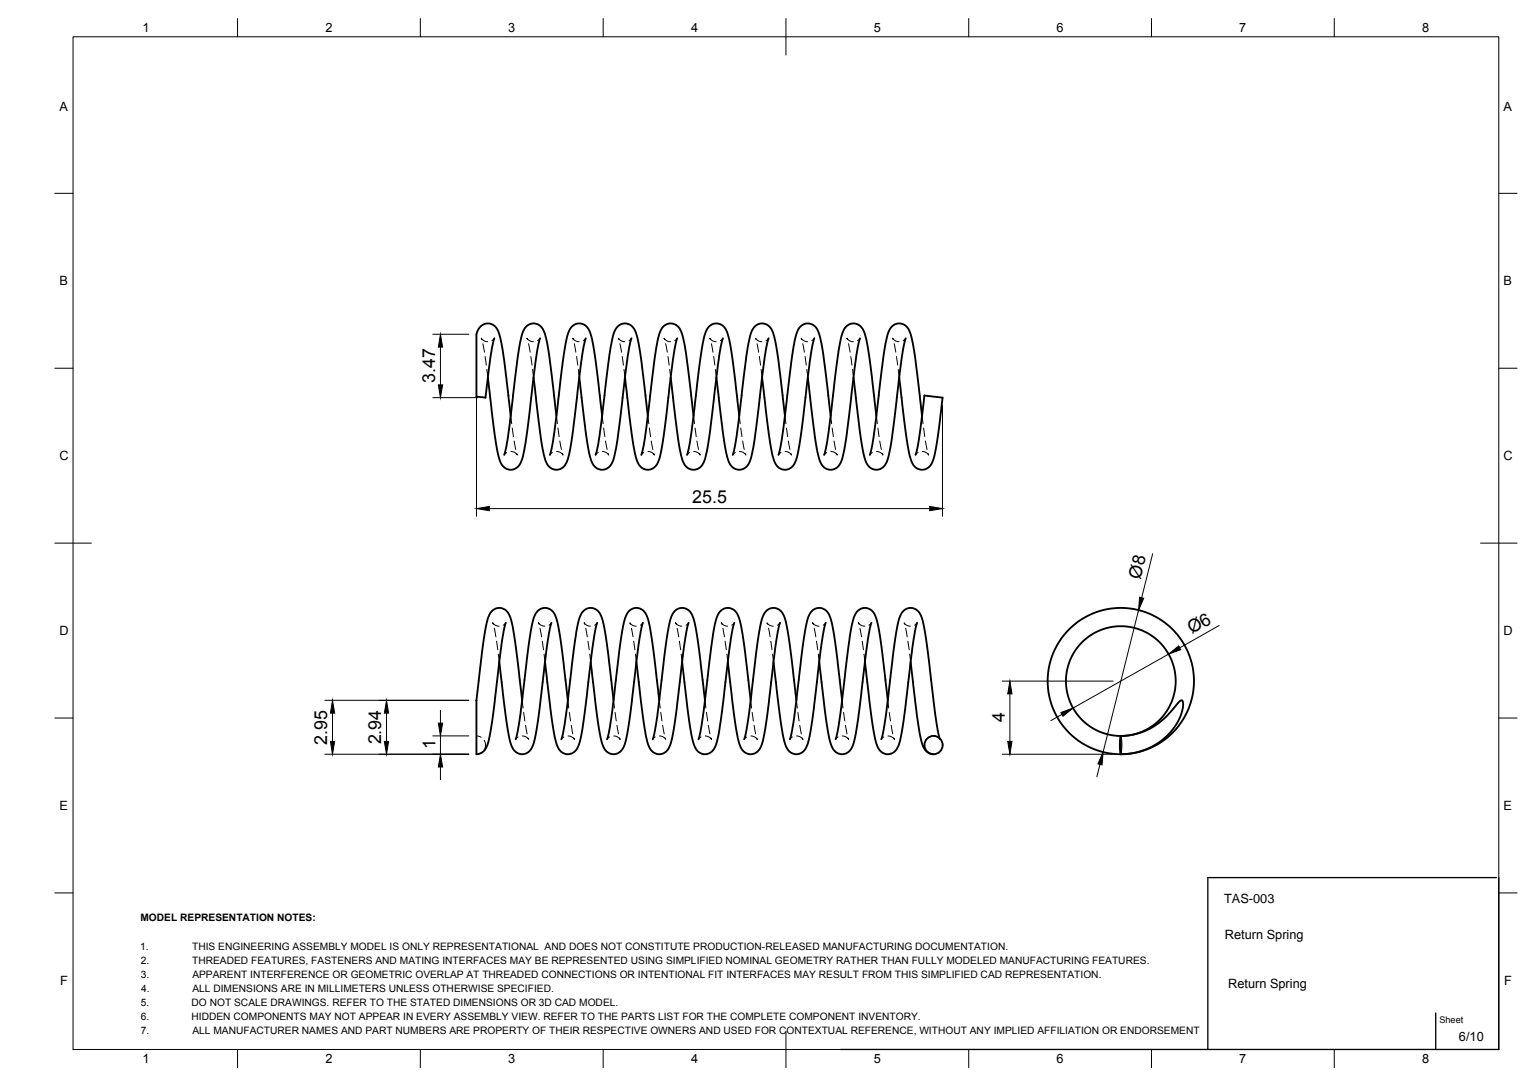
ISO-10303-21;
HEADER;
/* Generated by software containing ST-Developer
 * from STEP Tools, Inc. (www.steptools.com) 
 */

FILE_DESCRIPTION(
/* description */ ('STEP AP214'),
/* implementation_level */ '2;1');

FILE_NAME(
/* name */ 'Return Spring.step',
/* time_stamp */ '2026-11-04T19:43:37-08:00',
/* author */ (''),
/* organization */ (''),
/* preprocessor_version */ 'ST-DEVELOPER v20.2',
/* originating_system */ 'Autodesk Translation Framework v15.17.0.0',
/* authorisation */ '');

FILE_SCHEMA (('AUTOMOTIVE_DESIGN { 1 0 10303 214 3 1 1 }'));
ENDSEC;

DATA;
#10=MECHANICAL_DESIGN_GEOMETRIC_PRESENTATION_REPRESENTATION('',(#118),#7627);
#91=(
BOUNDED_CURVE()
B_SPLINE_CURVE(2,(#5252,#5253,#5254,#5255,#5256,#5257,#5258,#5259,#5260,
#5261,#5262,#5263,#5264,#5265,#5266,#5267,#5268,#5269,#5270,#5271,#5272,
#5273,#5274,#5275,#5276,#5277,#5278,#5279,#5280,#5281,#5282,#5283,#5284,
#5285,#5286,#5287,#5288,#5289,#5290,#5291,#5292,#5293,#5294,#5295,#5296,
#5297,#5298,#5299,#5300,#5301,#5302,#5303,#5304,#5305,#5306,#5307,#5308,
#5309,#5310,#5311,#5312,#5313,#5314,#5315,#5316,#5317,#5318,#5319,#5320,
#5321,#5322,#5323,#5324,#5325,#5326,#5327,#5328,#5329,#5330,#5331,#5332,
#5333,#5334,#5335,#5336,#5337,#5338,#5339,#5340,#5341,#5342,#5343,#5344,
#5345,#5346,#5347,#5348,#5349,#5350,#5351,#5352,#5353,#5354,#5355,#5356,
#5357,#5358,#5359,#5360,#5361,#5362,#5363,#5364,#5365,#5366,#5367,#5368,
#5369,#5370,#5371,#5372,#5373,#5374,#5375,#5376,#5377,#5378,#5379,#5380,
#5381,#5382,#5383,#5384,#5385,#5386,#5387,#5388,#5389,#5390,#5391,#5392,
#5393,#5394,#5395,#5396,#5397,#5398,#5399,#5400,#5401,#5402,#5403,#5404,
#5405,#5406,#5407,#5408,#5409,#5410,#5411,#5412,#5413,#5414,#5415,#5416,
#5417,#5418,#5419,#5420,#5421,#5422,#5423,#5424,#5425,#5426,#5427,#5428,
#5429,#5430,#5431,#5432,#5433,#5434,#5435,#5436,#5437,#5438,#5439,#5440,
#5441,#5442,#5443,#5444,#5445,#5446,#5447,#5448,#5449,#5450),
 .UNSPECIFIED.,.F.,.F.)
B_SPLINE_CURVE_WITH_KNOTS((3,2,2,2,2,2,2,2,2,2,2,2,2,2,2,2,2,2,2,2,2,2,
2,2,2,2,2,2,2,2,2,2,2,2,2,2,2,2,2,2,2,2,2,2,2,2,2,2,2,2,2,2,2,2,2,2,2,2,
2,2,2,2,2,2,2,2,2,2,2,2,2,2,2,2,2,2,2,2,2,2,2,2,2,2,2,2,2,2,2,2,2,2,2,2,
2,2,2,2,2,3),(0.0198656835159411,0.02,0.03,0.04,0.05,0.06,0.07,0.08,0.09,
0.1,0.11,0.12,0.13,0.14,0.15,0.16,0.17,0.18,0.19,0.2,0.21,0.22,0.23,0.24,
0.25,0.26,0.27,0.28,0.29,0.3,0.31,0.32,0.33,0.34,0.35,0.36,0.37,0.38,0.39,
0.4,0.41,0.42,0.43,0.44,0.45,0.46,0.47,0.48,0.49,0.5,0.51,0.52,0.53,0.54,
0.55,0.56,0.57,0.58,0.59,0.6,0.61,0.62,0.63,0.64,0.65,0.66,0.67,0.68,0.69,
0.7,0.71,0.72,0.73,0.74,0.75,0.76,0.77,0.78,0.79,0.8,0.81,0.82,0.83,0.84,
0.85,0.86,0.87,0.88,0.89,0.9,0.91,0.92,0.93,0.94,0.95,0.96,0.97,0.98,0.99,
1.),.UNSPECIFIED.)
CURVE()
GEOMETRIC_REPRESENTATION_ITEM()
RATIONAL_B_SPLINE_CURVE((0.998702876377649,0.999342608335117,1.,0.951056516295154,
1.,0.951056516295154,1.,0.951056516295154,1.,0.951056516295154,1.,0.951056516295154,
1.,0.951056516295154,1.,0.951056516295154,1.,0.951056516295154,1.,0.951056516295154,
1.,0.951056516295154,1.,0.951056516295154,1.,0.951056516295154,1.,0.951056516295154,
1.,0.951056516295154,1.,0.951056516295154,1.,0.951056516295154,1.,0.951056516295154,
1.,0.951056516295154,1.,0.951056516295154,1.,0.951056516295154,1.,0.951056516295154,
1.,0.951056516295154,1.,0.951056516295154,1.,0.951056516295154,1.,0.951056516295154,
1.,0.951056516295154,1.,0.951056516295154,1.,0.951056516295154,1.,0.951056516295154,
1.,0.951056516295154,1.,0.951056516295154,1.,0.951056516295154,1.,0.951056516295154,
1.,0.951056516295154,1.,0.951056516295154,1.,0.951056516295154,1.,0.951056516295154,
1.,0.951056516295154,1.,0.951056516295154,1.,0.951056516295154,1.,0.951056516295154,
1.,0.951056516295154,1.,0.951056516295154,1.,0.951056516295154,1.,0.951056516295154,
1.,0.951056516295154,1.,0.951056516295154,1.,0.951056516295154,1.,0.951056516295154,
1.,0.951056516295154,1.,0.951056516295154,1.,0.951056516295154,1.,0.951056516295154,
1.,0.951056516295154,1.,0.951056516295154,1.,0.951056516295154,1.,0.951056516295154,
1.,0.951056516295154,1.,0.951056516295154,1.,0.951056516295154,1.,0.951056516295154,
1.,0.951056516295154,1.,0.951056516295154,1.,0.951056516295154,1.,0.951056516295154,
1.,0.951056516295154,1.,0.951056516295154,1.,0.951056516295154,1.,0.951056516295154,
1.,0.951056516295154,1.,0.951056516295154,1.,0.951056516295154,1.,0.951056516295154,
1.,0.951056516295154,1.,0.951056516295154,1.,0.951056516295154,1.,0.951056516295154,
1.,0.951056516295154,1.,0.951056516295154,1.,0.951056516295154,1.,0.951056516295154,
1.,0.951056516295154,1.,0.951056516295154,1.,0.951056516295154,1.,0.951056516295154,
1.,0.951056516295154,1.,0.951056516295154,1.,0.951056516295154,1.,0.951056516295154,
1.,0.951056516295154,1.,0.951056516295154,1.,0.951056516295154,1.,0.951056516295154,
1.,0.951056516295154,1.,0.951056516295154,1.,0.951056516295154,1.,0.951056516295154,
1.,0.951056516295154,1.))
REPRESENTATION_ITEM('')
);
#92=(
BOUNDED_CURVE()
B_SPLINE_CURVE(2,(#5454,#5455,#5456,#5457,#5458,#5459,#5460,#5461,#5462,
#5463,#5464,#5465,#5466,#5467,#5468,#5469,#5470,#5471,#5472,#5473,#5474,
#5475,#5476,#5477,#5478,#5479,#5480,#5481,#5482,#5483,#5484,#5485,#5486,
#5487,#5488,#5489,#5490,#5491,#5492,#5493,#5494,#5495,#5496,#5497,#5498,
#5499,#5500,#5501,#5502,#5503,#5504,#5505,#5506,#5507,#5508,#5509,#5510,
#5511,#5512,#5513,#5514,#5515,#5516,#5517,#5518,#5519,#5520,#5521,#5522,
#5523,#5524,#5525,#5526,#5527,#5528,#5529,#5530,#5531,#5532,#5533,#5534,
#5535,#5536,#5537,#5538,#5539,#5540,#5541,#5542,#5543,#5544,#5545,#5546,
#5547,#5548,#5549,#5550,#5551,#5552,#5553,#5554,#5555,#5556,#5557,#5558,
#5559,#5560,#5561,#5562,#5563,#5564,#5565,#5566,#5567,#5568,#5569,#5570,
#5571,#5572,#5573,#5574,#5575,#5576,#5577,#5578,#5579,#5580,#5581,#5582,
#5583,#5584,#5585,#5586,#5587,#5588,#5589,#5590,#5591,#5592,#5593,#5594,
#5595,#5596,#5597,#5598,#5599,#5600,#5601,#5602,#5603,#5604,#5605,#5606,
#5607,#5608,#5609,#5610,#5611,#5612,#5613,#5614,#5615,#5616,#5617,#5618,
#5619,#5620,#5621,#5622,#5623,#5624,#5625,#5626,#5627,#5628,#5629,#5630,
#5631,#5632,#5633,#5634,#5635,#5636,#5637,#5638,#5639,#5640,#5641,#5642,
#5643,#5644,#5645,#5646,#5647,#5648,#5649,#5650,#5651,#5652,#5653,#5654),
 .UNSPECIFIED.,.F.,.F.)
B_SPLINE_CURVE_WITH_KNOTS((3,2,2,2,2,2,2,2,2,2,2,2,2,2,2,2,2,2,2,2,2,2,
2,2,2,2,2,2,2,2,2,2,2,2,2,2,2,2,2,2,2,2,2,2,2,2,2,2,2,2,2,2,2,2,2,2,2,2,
2,2,2,2,2,2,2,2,2,2,2,2,2,2,2,2,2,2,2,2,2,2,2,2,2,2,2,2,2,2,2,2,2,2,2,2,
2,2,2,2,2,2,3),(0.,0.01,0.02,0.03,0.04,0.05,0.06,0.07,0.08,0.09,0.1,0.11,
0.12,0.13,0.14,0.15,0.16,0.17,0.18,0.19,0.2,0.21,0.22,0.23,0.24,0.25,0.26,
0.27,0.28,0.29,0.3,0.31,0.32,0.33,0.34,0.35,0.36,0.37,0.38,0.39,0.4,0.41,
0.42,0.43,0.44,0.45,0.46,0.47,0.48,0.49,0.5,0.51,0.52,0.53,0.54,0.55,0.56,
0.57,0.58,0.59,0.6,0.61,0.62,0.63,0.64,0.65,0.66,0.67,0.68,0.69,0.7,0.71,
0.72,0.73,0.74,0.75,0.76,0.77,0.78,0.79,0.8,0.81,0.82,0.83,0.84,0.85,0.86,
0.87,0.88,0.89,0.9,0.91,0.92,0.93,0.94,0.95,0.96,0.97,0.98,0.99,1.),
 .UNSPECIFIED.)
CURVE()
GEOMETRIC_REPRESENTATION_ITEM()
RATIONAL_B_SPLINE_CURVE((1.,0.951056516295154,1.,0.951056516295154,1.,0.951056516295154,
1.,0.951056516295154,1.,0.951056516295154,1.,0.951056516295154,1.,0.951056516295154,
1.,0.951056516295154,1.,0.951056516295154,1.,0.951056516295154,1.,0.951056516295154,
1.,0.951056516295154,1.,0.951056516295154,1.,0.951056516295154,1.,0.951056516295154,
1.,0.951056516295154,1.,0.951056516295154,1.,0.951056516295154,1.,0.951056516295154,
1.,0.951056516295154,1.,0.951056516295154,1.,0.951056516295154,1.,0.951056516295154,
1.,0.951056516295154,1.,0.951056516295154,1.,0.951056516295154,1.,0.951056516295154,
1.,0.951056516295154,1.,0.951056516295154,1.,0.951056516295154,1.,0.951056516295154,
1.,0.951056516295154,1.,0.951056516295154,1.,0.951056516295154,1.,0.951056516295154,
1.,0.951056516295154,1.,0.951056516295154,1.,0.951056516295154,1.,0.951056516295154,
1.,0.951056516295154,1.,0.951056516295154,1.,0.951056516295154,1.,0.951056516295154,
1.,0.951056516295154,1.,0.951056516295154,1.,0.951056516295154,1.,0.951056516295154,
1.,0.951056516295154,1.,0.951056516295154,1.,0.951056516295154,1.,0.951056516295154,
1.,0.951056516295154,1.,0.951056516295154,1.,0.951056516295154,1.,0.951056516295154,
1.,0.951056516295154,1.,0.951056516295154,1.,0.951056516295154,1.,0.951056516295154,
1.,0.951056516295154,1.,0.951056516295154,1.,0.951056516295154,1.,0.951056516295154,
1.,0.951056516295154,1.,0.951056516295154,1.,0.951056516295154,1.,0.951056516295154,
1.,0.951056516295154,1.,0.951056516295154,1.,0.951056516295154,1.,0.951056516295154,
1.,0.951056516295154,1.,0.951056516295154,1.,0.951056516295154,1.,0.951056516295154,
1.,0.951056516295154,1.,0.951056516295154,1.,0.951056516295154,1.,0.951056516295154,
1.,0.951056516295154,1.,0.951056516295154,1.,0.951056516295154,1.,0.951056516295154,
1.,0.951056516295154,1.,0.951056516295154,1.,0.951056516295154,1.,0.951056516295154,
1.,0.951056516295154,1.,0.951056516295154,1.,0.951056516295154,1.,0.951056516295154,
1.,0.951056516295154,1.,0.951056516295154,1.,0.951056516295154,1.,0.951056516295154,
1.,0.951056516295154,1.,0.951056516295154,1.,0.951056516295154,1.,0.951056516295154,
1.,0.951056516295154,1.))
REPRESENTATION_ITEM('')
);
#93=B_SPLINE_CURVE_WITH_KNOTS('',3,(#5233,#5234,#5235,#5236,#5237,#5238,
#5239,#5240,#5241,#5242,#5243,#5244,#5245,#5246,#5247,#5248,#5249,#5250),
 .UNSPECIFIED.,.F.,.F.,(4,2,2,2,2,2,2,2,4),(1.00001181076875E-6,0.00157652680691075,
0.00330831465659758,0.00743558655671621,0.0176553842502255,0.0434588790338826,
0.0717527150596022,0.0885002828939342,0.104340792550165),.UNSPECIFIED.);
#94=B_SPLINE_CURVE_WITH_KNOTS('',3,(#7069,#7070,#7071,#7072,#7073,#7074,
#7075,#7076,#7077,#7078,#7079,#7080,#7081,#7082,#7083,#7084,#7085,#7086),
 .UNSPECIFIED.,.F.,.F.,(4,2,2,2,2,2,2,2,4),(0.,0.132188814767311,0.250674887289718,
0.391272166110131,0.552836235371939,0.655950520994649,0.689957274574409,
0.701859173270786,0.711834218003037),.UNSPECIFIED.);
#95=(
BOUNDED_SURFACE()
B_SPLINE_SURFACE(3,2,((#3824,#3825,#3826,#3827,#3828,#3829,#3830,#3831,
#3832,#3833,#3834,#3835,#3836,#3837,#3838,#3839,#3840,#3841,#3842,#3843,
#3844,#3845,#3846,#3847,#3848,#3849,#3850,#3851,#3852,#3853,#3854,#3855,
#3856,#3857,#3858,#3859,#3860,#3861,#3862,#3863,#3864,#3865,#3866,#3867,
#3868,#3869,#3870,#3871,#3872,#3873,#3874,#3875,#3876,#3877,#3878,#3879,
#3880,#3881,#3882,#3883,#3884,#3885,#3886,#3887,#3888,#3889,#3890,#3891,
#3892,#3893,#3894,#3895,#3896,#3897,#3898,#3899,#3900,#3901,#3902,#3903,
#3904,#3905,#3906,#3907,#3908,#3909,#3910,#3911,#3912,#3913,#3914,#3915,
#3916,#3917,#3918,#3919,#3920,#3921,#3922,#3923,#3924,#3925,#3926,#3927,
#3928,#3929,#3930,#3931,#3932,#3933,#3934,#3935,#3936,#3937,#3938,#3939,
#3940,#3941,#3942,#3943,#3944,#3945,#3946,#3947,#3948,#3949,#3950,#3951,
#3952,#3953,#3954,#3955,#3956,#3957,#3958,#3959,#3960,#3961,#3962,#3963,
#3964,#3965,#3966,#3967,#3968,#3969,#3970,#3971,#3972,#3973,#3974,#3975,
#3976,#3977,#3978,#3979,#3980,#3981,#3982,#3983,#3984,#3985,#3986,#3987,
#3988,#3989,#3990,#3991,#3992,#3993,#3994,#3995,#3996,#3997,#3998,#3999,
#4000,#4001,#4002,#4003,#4004,#4005,#4006,#4007,#4008,#4009,#4010,#4011,
#4012,#4013,#4014,#4015,#4016,#4017,#4018,#4019,#4020,#4021,#4022,#4023,
#4024),(#4025,#4026,#4027,#4028,#4029,#4030,#4031,#4032,#4033,#4034,#4035,
#4036,#4037,#4038,#4039,#4040,#4041,#4042,#4043,#4044,#4045,#4046,#4047,
#4048,#4049,#4050,#4051,#4052,#4053,#4054,#4055,#4056,#4057,#4058,#4059,
#4060,#4061,#4062,#4063,#4064,#4065,#4066,#4067,#4068,#4069,#4070,#4071,
#4072,#4073,#4074,#4075,#4076,#4077,#4078,#4079,#4080,#4081,#4082,#4083,
#4084,#4085,#4086,#4087,#4088,#4089,#4090,#4091,#4092,#4093,#4094,#4095,
#4096,#4097,#4098,#4099,#4100,#4101,#4102,#4103,#4104,#4105,#4106,#4107,
#4108,#4109,#4110,#4111,#4112,#4113,#4114,#4115,#4116,#4117,#4118,#4119,
#4120,#4121,#4122,#4123,#4124,#4125,#4126,#4127,#4128,#4129,#4130,#4131,
#4132,#4133,#4134,#4135,#4136,#4137,#4138,#4139,#4140,#4141,#4142,#4143,
#4144,#4145,#4146,#4147,#4148,#4149,#4150,#4151,#4152,#4153,#4154,#4155,
#4156,#4157,#4158,#4159,#4160,#4161,#4162,#4163,#4164,#4165,#4166,#4167,
#4168,#4169,#4170,#4171,#4172,#4173,#4174,#4175,#4176,#4177,#4178,#4179,
#4180,#4181,#4182,#4183,#4184,#4185,#4186,#4187,#4188,#4189,#4190,#4191,
#4192,#4193,#4194,#4195,#4196,#4197,#4198,#4199,#4200,#4201,#4202,#4203,
#4204,#4205,#4206,#4207,#4208,#4209,#4210,#4211,#4212,#4213,#4214,#4215,
#4216,#4217,#4218,#4219,#4220,#4221,#4222,#4223,#4224,#4225),(#4226,#4227,
#4228,#4229,#4230,#4231,#4232,#4233,#4234,#4235,#4236,#4237,#4238,#4239,
#4240,#4241,#4242,#4243,#4244,#4245,#4246,#4247,#4248,#4249,#4250,#4251,
#4252,#4253,#4254,#4255,#4256,#4257,#4258,#4259,#4260,#4261,#4262,#4263,
#4264,#4265,#4266,#4267,#4268,#4269,#4270,#4271,#4272,#4273,#4274,#4275,
#4276,#4277,#4278,#4279,#4280,#4281,#4282,#4283,#4284,#4285,#4286,#4287,
#4288,#4289,#4290,#4291,#4292,#4293,#4294,#4295,#4296,#4297,#4298,#4299,
#4300,#4301,#4302,#4303,#4304,#4305,#4306,#4307,#4308,#4309,#4310,#4311,
#4312,#4313,#4314,#4315,#4316,#4317,#4318,#4319,#4320,#4321,#4322,#4323,
#4324,#4325,#4326,#4327,#4328,#4329,#4330,#4331,#4332,#4333,#4334,#4335,
#4336,#4337,#4338,#4339,#4340,#4341,#4342,#4343,#4344,#4345,#4346,#4347,
#4348,#4349,#4350,#4351,#4352,#4353,#4354,#4355,#4356,#4357,#4358,#4359,
#4360,#4361,#4362,#4363,#4364,#4365,#4366,#4367,#4368,#4369,#4370,#4371,
#4372,#4373,#4374,#4375,#4376,#4377,#4378,#4379,#4380,#4381,#4382,#4383,
#4384,#4385,#4386,#4387,#4388,#4389,#4390,#4391,#4392,#4393,#4394,#4395,
#4396,#4397,#4398,#4399,#4400,#4401,#4402,#4403,#4404,#4405,#4406,#4407,
#4408,#4409,#4410,#4411,#4412,#4413,#4414,#4415,#4416,#4417,#4418,#4419,
#4420,#4421,#4422,#4423,#4424,#4425,#4426),(#4427,#4428,#4429,#4430,#4431,
#4432,#4433,#4434,#4435,#4436,#4437,#4438,#4439,#4440,#4441,#4442,#4443,
#4444,#4445,#4446,#4447,#4448,#4449,#4450,#4451,#4452,#4453,#4454,#4455,
#4456,#4457,#4458,#4459,#4460,#4461,#4462,#4463,#4464,#4465,#4466,#4467,
#4468,#4469,#4470,#4471,#4472,#4473,#4474,#4475,#4476,#4477,#4478,#4479,
#4480,#4481,#4482,#4483,#4484,#4485,#4486,#4487,#4488,#4489,#4490,#4491,
#4492,#4493,#4494,#4495,#4496,#4497,#4498,#4499,#4500,#4501,#4502,#4503,
#4504,#4505,#4506,#4507,#4508,#4509,#4510,#4511,#4512,#4513,#4514,#4515,
#4516,#4517,#4518,#4519,#4520,#4521,#4522,#4523,#4524,#4525,#4526,#4527,
#4528,#4529,#4530,#4531,#4532,#4533,#4534,#4535,#4536,#4537,#4538,#4539,
#4540,#4541,#4542,#4543,#4544,#4545,#4546,#4547,#4548,#4549,#4550,#4551,
#4552,#4553,#4554,#4555,#4556,#4557,#4558,#4559,#4560,#4561,#4562,#4563,
#4564,#4565,#4566,#4567,#4568,#4569,#4570,#4571,#4572,#4573,#4574,#4575,
#4576,#4577,#4578,#4579,#4580,#4581,#4582,#4583,#4584,#4585,#4586,#4587,
#4588,#4589,#4590,#4591,#4592,#4593,#4594,#4595,#4596,#4597,#4598,#4599,
#4600,#4601,#4602,#4603,#4604,#4605,#4606,#4607,#4608,#4609,#4610,#4611,
#4612,#4613,#4614,#4615,#4616,#4617,#4618,#4619,#4620,#4621,#4622,#4623,
#4624,#4625,#4626,#4627),(#4628,#4629,#4630,#4631,#4632,#4633,#4634,#4635,
#4636,#4637,#4638,#4639,#4640,#4641,#4642,#4643,#4644,#4645,#4646,#4647,
#4648,#4649,#4650,#4651,#4652,#4653,#4654,#4655,#4656,#4657,#4658,#4659,
#4660,#4661,#4662,#4663,#4664,#4665,#4666,#4667,#4668,#4669,#4670,#4671,
#4672,#4673,#4674,#4675,#4676,#4677,#4678,#4679,#4680,#4681,#4682,#4683,
#4684,#4685,#4686,#4687,#4688,#4689,#4690,#4691,#4692,#4693,#4694,#4695,
#4696,#4697,#4698,#4699,#4700,#4701,#4702,#4703,#4704,#4705,#4706,#4707,
#4708,#4709,#4710,#4711,#4712,#4713,#4714,#4715,#4716,#4717,#4718,#4719,
#4720,#4721,#4722,#4723,#4724,#4725,#4726,#4727,#4728,#4729,#4730,#4731,
#4732,#4733,#4734,#4735,#4736,#4737,#4738,#4739,#4740,#4741,#4742,#4743,
#4744,#4745,#4746,#4747,#4748,#4749,#4750,#4751,#4752,#4753,#4754,#4755,
#4756,#4757,#4758,#4759,#4760,#4761,#4762,#4763,#4764,#4765,#4766,#4767,
#4768,#4769,#4770,#4771,#4772,#4773,#4774,#4775,#4776,#4777,#4778,#4779,
#4780,#4781,#4782,#4783,#4784,#4785,#4786,#4787,#4788,#4789,#4790,#4791,
#4792,#4793,#4794,#4795,#4796,#4797,#4798,#4799,#4800,#4801,#4802,#4803,
#4804,#4805,#4806,#4807,#4808,#4809,#4810,#4811,#4812,#4813,#4814,#4815,
#4816,#4817,#4818,#4819,#4820,#4821,#4822,#4823,#4824,#4825,#4826,#4827,
#4828),(#4829,#4830,#4831,#4832,#4833,#4834,#4835,#4836,#4837,#4838,#4839,
#4840,#4841,#4842,#4843,#4844,#4845,#4846,#4847,#4848,#4849,#4850,#4851,
#4852,#4853,#4854,#4855,#4856,#4857,#4858,#4859,#4860,#4861,#4862,#4863,
#4864,#4865,#4866,#4867,#4868,#4869,#4870,#4871,#4872,#4873,#4874,#4875,
#4876,#4877,#4878,#4879,#4880,#4881,#4882,#4883,#4884,#4885,#4886,#4887,
#4888,#4889,#4890,#4891,#4892,#4893,#4894,#4895,#4896,#4897,#4898,#4899,
#4900,#4901,#4902,#4903,#4904,#4905,#4906,#4907,#4908,#4909,#4910,#4911,
#4912,#4913,#4914,#4915,#4916,#4917,#4918,#4919,#4920,#4921,#4922,#4923,
#4924,#4925,#4926,#4927,#4928,#4929,#4930,#4931,#4932,#4933,#4934,#4935,
#4936,#4937,#4938,#4939,#4940,#4941,#4942,#4943,#4944,#4945,#4946,#4947,
#4948,#4949,#4950,#4951,#4952,#4953,#4954,#4955,#4956,#4957,#4958,#4959,
#4960,#4961,#4962,#4963,#4964,#4965,#4966,#4967,#4968,#4969,#4970,#4971,
#4972,#4973,#4974,#4975,#4976,#4977,#4978,#4979,#4980,#4981,#4982,#4983,
#4984,#4985,#4986,#4987,#4988,#4989,#4990,#4991,#4992,#4993,#4994,#4995,
#4996,#4997,#4998,#4999,#5000,#5001,#5002,#5003,#5004,#5005,#5006,#5007,
#5008,#5009,#5010,#5011,#5012,#5013,#5014,#5015,#5016,#5017,#5018,#5019,
#5020,#5021,#5022,#5023,#5024,#5025,#5026,#5027,#5028,#5029),(#5030,#5031,
#5032,#5033,#5034,#5035,#5036,#5037,#5038,#5039,#5040,#5041,#5042,#5043,
#5044,#5045,#5046,#5047,#5048,#5049,#5050,#5051,#5052,#5053,#5054,#5055,
#5056,#5057,#5058,#5059,#5060,#5061,#5062,#5063,#5064,#5065,#5066,#5067,
#5068,#5069,#5070,#5071,#5072,#5073,#5074,#5075,#5076,#5077,#5078,#5079,
#5080,#5081,#5082,#5083,#5084,#5085,#5086,#5087,#5088,#5089,#5090,#5091,
#5092,#5093,#5094,#5095,#5096,#5097,#5098,#5099,#5100,#5101,#5102,#5103,
#5104,#5105,#5106,#5107,#5108,#5109,#5110,#5111,#5112,#5113,#5114,#5115,
#5116,#5117,#5118,#5119,#5120,#5121,#5122,#5123,#5124,#5125,#5126,#5127,
#5128,#5129,#5130,#5131,#5132,#5133,#5134,#5135,#5136,#5137,#5138,#5139,
#5140,#5141,#5142,#5143,#5144,#5145,#5146,#5147,#5148,#5149,#5150,#5151,
#5152,#5153,#5154,#5155,#5156,#5157,#5158,#5159,#5160,#5161,#5162,#5163,
#5164,#5165,#5166,#5167,#5168,#5169,#5170,#5171,#5172,#5173,#5174,#5175,
#5176,#5177,#5178,#5179,#5180,#5181,#5182,#5183,#5184,#5185,#5186,#5187,
#5188,#5189,#5190,#5191,#5192,#5193,#5194,#5195,#5196,#5197,#5198,#5199,
#5200,#5201,#5202,#5203,#5204,#5205,#5206,#5207,#5208,#5209,#5210,#5211,
#5212,#5213,#5214,#5215,#5216,#5217,#5218,#5219,#5220,#5221,#5222,#5223,
#5224,#5225,#5226,#5227,#5228,#5229,#5230)),.UNSPECIFIED.,.T.,.F.,.F.)
B_SPLINE_SURFACE_WITH_KNOTS((4,3,4),(3,2,2,2,2,2,2,2,2,2,2,2,2,2,2,2,2,
2,2,2,2,2,2,2,2,2,2,2,2,2,2,2,2,2,2,2,2,2,2,2,2,2,2,2,2,2,2,2,2,2,2,2,2,
2,2,2,2,2,2,2,2,2,2,2,2,2,2,2,2,2,2,2,2,2,2,2,2,2,2,2,2,2,2,2,2,2,2,2,2,
2,2,2,2,2,2,2,2,2,2,2,3),(0.,0.5,1.),(0.,0.01,0.02,0.03,0.04,0.05,0.06,
0.07,0.08,0.09,0.1,0.11,0.12,0.13,0.14,0.15,0.16,0.17,0.18,0.19,0.2,0.21,
0.22,0.23,0.24,0.25,0.26,0.27,0.28,0.29,0.3,0.31,0.32,0.33,0.34,0.35,0.36,
0.37,0.38,0.39,0.4,0.41,0.42,0.43,0.44,0.45,0.46,0.47,0.48,0.49,0.5,0.51,
0.52,0.53,0.54,0.55,0.56,0.57,0.58,0.59,0.6,0.61,0.62,0.63,0.64,0.65,0.66,
0.67,0.68,0.69,0.7,0.71,0.72,0.73,0.74,0.75,0.76,0.77,0.78,0.79,0.8,0.81,
0.82,0.83,0.84,0.85,0.86,0.87,0.88,0.89,0.9,0.91,0.92,0.93,0.94,0.95,0.96,
0.97,0.98,0.99,1.),.UNSPECIFIED.)
GEOMETRIC_REPRESENTATION_ITEM()
RATIONAL_B_SPLINE_SURFACE(((1.,0.951056516295154,1.,0.951056516295154,1.,
0.951056516295154,1.,0.951056516295154,1.,0.951056516295154,1.,0.951056516295154,
1.,0.951056516295154,1.,0.951056516295154,1.,0.951056516295154,1.,0.951056516295154,
1.,0.951056516295154,1.,0.951056516295154,1.,0.951056516295154,1.,0.951056516295154,
1.,0.951056516295154,1.,0.951056516295154,1.,0.951056516295154,1.,0.951056516295154,
1.,0.951056516295154,1.,0.951056516295154,1.,0.951056516295154,1.,0.951056516295154,
1.,0.951056516295154,1.,0.951056516295154,1.,0.951056516295154,1.,0.951056516295154,
1.,0.951056516295154,1.,0.951056516295154,1.,0.951056516295154,1.,0.951056516295154,
1.,0.951056516295154,1.,0.951056516295154,1.,0.951056516295154,1.,0.951056516295154,
1.,0.951056516295154,1.,0.951056516295154,1.,0.951056516295154,1.,0.951056516295154,
1.,0.951056516295154,1.,0.951056516295154,1.,0.951056516295154,1.,0.951056516295154,
1.,0.951056516295154,1.,0.951056516295154,1.,0.951056516295154,1.,0.951056516295154,
1.,0.951056516295154,1.,0.951056516295154,1.,0.951056516295154,1.,0.951056516295154,
1.,0.951056516295154,1.,0.951056516295154,1.,0.951056516295154,1.,0.951056516295154,
1.,0.951056516295154,1.,0.951056516295154,1.,0.951056516295154,1.,0.951056516295154,
1.,0.951056516295154,1.,0.951056516295154,1.,0.951056516295154,1.,0.951056516295154,
1.,0.951056516295154,1.,0.951056516295154,1.,0.951056516295154,1.,0.951056516295154,
1.,0.951056516295154,1.,0.951056516295154,1.,0.951056516295154,1.,0.951056516295154,
1.,0.951056516295154,1.,0.951056516295154,1.,0.951056516295154,1.,0.951056516295154,
1.,0.951056516295154,1.,0.951056516295154,1.,0.951056516295154,1.,0.951056516295154,
1.,0.951056516295154,1.,0.951056516295154,1.,0.951056516295154,1.,0.951056516295154,
1.,0.951056516295154,1.,0.951056516295154,1.,0.951056516295154,1.,0.951056516295154,
1.,0.951056516295154,1.,0.951056516295154,1.,0.951056516295154,1.,0.951056516295154,
1.,0.951056516295154,1.,0.951056516295154,1.,0.951056516295154,1.,0.951056516295154,
1.,0.951056516295154,1.,0.951056516295154,1.,0.951056516295154,1.,0.951056516295154,
1.,0.951056516295154,1.,0.951056516295154,1.),(0.333333333333333,0.317018838765051,
0.333333333333333,0.317018838765051,0.333333333333333,0.317018838765051,
0.333333333333333,0.317018838765051,0.333333333333333,0.317018838765051,
0.333333333333333,0.317018838765051,0.333333333333333,0.317018838765051,
0.333333333333333,0.317018838765051,0.333333333333333,0.317018838765051,
0.333333333333333,0.317018838765051,0.333333333333333,0.317018838765051,
0.333333333333333,0.317018838765051,0.333333333333333,0.317018838765051,
0.333333333333333,0.317018838765051,0.333333333333333,0.317018838765051,
0.333333333333333,0.317018838765051,0.333333333333333,0.317018838765051,
0.333333333333333,0.317018838765051,0.333333333333333,0.317018838765051,
0.333333333333333,0.317018838765051,0.333333333333333,0.317018838765051,
0.333333333333333,0.317018838765051,0.333333333333333,0.317018838765051,
0.333333333333333,0.317018838765051,0.333333333333333,0.317018838765051,
0.333333333333333,0.317018838765051,0.333333333333333,0.317018838765051,
0.333333333333333,0.317018838765051,0.333333333333333,0.317018838765051,
0.333333333333333,0.317018838765051,0.333333333333333,0.317018838765051,
0.333333333333333,0.317018838765051,0.333333333333333,0.317018838765051,
0.333333333333333,0.317018838765051,0.333333333333333,0.317018838765051,
0.333333333333333,0.317018838765051,0.333333333333333,0.317018838765051,
0.333333333333333,0.317018838765051,0.333333333333333,0.317018838765051,
0.333333333333333,0.317018838765051,0.333333333333333,0.317018838765051,
0.333333333333333,0.317018838765051,0.333333333333333,0.317018838765051,
0.333333333333333,0.317018838765051,0.333333333333333,0.317018838765051,
0.333333333333333,0.317018838765051,0.333333333333333,0.317018838765051,
0.333333333333333,0.317018838765051,0.333333333333333,0.317018838765051,
0.333333333333333,0.317018838765051,0.333333333333333,0.317018838765051,
0.333333333333333,0.317018838765051,0.333333333333333,0.317018838765051,
0.333333333333333,0.317018838765051,0.333333333333333,0.317018838765051,
0.333333333333333,0.317018838765051,0.333333333333333,0.317018838765051,
0.333333333333333,0.317018838765051,0.333333333333333,0.317018838765051,
0.333333333333333,0.317018838765051,0.333333333333333,0.317018838765051,
0.333333333333333,0.317018838765051,0.333333333333333,0.317018838765051,
0.333333333333333,0.317018838765051,0.333333333333333,0.317018838765051,
0.333333333333333,0.317018838765051,0.333333333333333,0.317018838765051,
0.333333333333333,0.317018838765051,0.333333333333333,0.317018838765051,
0.333333333333333,0.317018838765051,0.333333333333333,0.317018838765051,
0.333333333333333,0.317018838765051,0.333333333333333,0.317018838765051,
0.333333333333333,0.317018838765051,0.333333333333333,0.317018838765051,
0.333333333333333,0.317018838765051,0.333333333333333,0.317018838765051,
0.333333333333333,0.317018838765051,0.333333333333333,0.317018838765051,
0.333333333333333,0.317018838765051,0.333333333333333,0.317018838765051,
0.333333333333333,0.317018838765051,0.333333333333333,0.317018838765051,
0.333333333333333,0.317018838765051,0.333333333333333,0.317018838765051,
0.333333333333333,0.317018838765051,0.333333333333333,0.317018838765051,
0.333333333333333,0.317018838765051,0.333333333333333,0.317018838765051,
0.333333333333333,0.317018838765051,0.333333333333333,0.317018838765051,
0.333333333333333,0.317018838765051,0.333333333333333,0.317018838765051,
0.333333333333333,0.317018838765051,0.333333333333333,0.317018838765051,
0.333333333333333,0.317018838765051,0.333333333333333,0.317018838765051,
0.333333333333333,0.317018838765051,0.333333333333333,0.317018838765051,
0.333333333333333,0.317018838765051,0.333333333333333),(0.333333333333333,
0.317018838765051,0.333333333333333,0.317018838765051,0.333333333333333,
0.317018838765051,0.333333333333333,0.317018838765051,0.333333333333333,
0.317018838765051,0.333333333333333,0.317018838765051,0.333333333333333,
0.317018838765051,0.333333333333333,0.317018838765051,0.333333333333333,
0.317018838765051,0.333333333333333,0.317018838765051,0.333333333333333,
0.317018838765051,0.333333333333333,0.317018838765051,0.333333333333333,
0.317018838765051,0.333333333333333,0.317018838765051,0.333333333333333,
0.317018838765051,0.333333333333333,0.317018838765051,0.333333333333333,
0.317018838765051,0.333333333333333,0.317018838765051,0.333333333333333,
0.317018838765051,0.333333333333333,0.317018838765051,0.333333333333333,
0.317018838765051,0.333333333333333,0.317018838765051,0.333333333333333,
0.317018838765051,0.333333333333333,0.317018838765051,0.333333333333333,
0.317018838765051,0.333333333333333,0.317018838765051,0.333333333333333,
0.317018838765051,0.333333333333333,0.317018838765051,0.333333333333333,
0.317018838765051,0.333333333333333,0.317018838765051,0.333333333333333,
0.317018838765051,0.333333333333333,0.317018838765051,0.333333333333333,
0.317018838765051,0.333333333333333,0.317018838765051,0.333333333333333,
0.317018838765051,0.333333333333333,0.317018838765051,0.333333333333333,
0.317018838765051,0.333333333333333,0.317018838765051,0.333333333333333,
0.317018838765051,0.333333333333333,0.317018838765051,0.333333333333333,
0.317018838765051,0.333333333333333,0.317018838765051,0.333333333333333,
0.317018838765051,0.333333333333333,0.317018838765051,0.333333333333333,
0.317018838765051,0.333333333333333,0.317018838765051,0.333333333333333,
0.317018838765051,0.333333333333333,0.317018838765051,0.333333333333333,
0.317018838765051,0.333333333333333,0.317018838765051,0.333333333333333,
0.317018838765051,0.333333333333333,0.317018838765051,0.333333333333333,
0.317018838765051,0.333333333333333,0.317018838765051,0.333333333333333,
0.317018838765051,0.333333333333333,0.317018838765051,0.333333333333333,
0.317018838765051,0.333333333333333,0.317018838765051,0.333333333333333,
0.317018838765051,0.333333333333333,0.317018838765051,0.333333333333333,
0.317018838765051,0.333333333333333,0.317018838765051,0.333333333333333,
0.317018838765051,0.333333333333333,0.317018838765051,0.333333333333333,
0.317018838765051,0.333333333333333,0.317018838765051,0.333333333333333,
0.317018838765051,0.333333333333333,0.317018838765051,0.333333333333333,
0.317018838765051,0.333333333333333,0.317018838765051,0.333333333333333,
0.317018838765051,0.333333333333333,0.317018838765051,0.333333333333333,
0.317018838765051,0.333333333333333,0.317018838765051,0.333333333333333,
0.317018838765051,0.333333333333333,0.317018838765051,0.333333333333333,
0.317018838765051,0.333333333333333,0.317018838765051,0.333333333333333,
0.317018838765051,0.333333333333333,0.317018838765051,0.333333333333333,
0.317018838765051,0.333333333333333,0.317018838765051,0.333333333333333,
0.317018838765051,0.333333333333333,0.317018838765051,0.333333333333333,
0.317018838765051,0.333333333333333,0.317018838765051,0.333333333333333,
0.317018838765051,0.333333333333333,0.317018838765051,0.333333333333333,
0.317018838765051,0.333333333333333,0.317018838765051,0.333333333333333,
0.317018838765051,0.333333333333333,0.317018838765051,0.333333333333333,
0.317018838765051,0.333333333333333,0.317018838765051,0.333333333333333,
0.317018838765051,0.333333333333333,0.317018838765051,0.333333333333333,
0.317018838765051,0.333333333333333,0.317018838765051,0.333333333333333,
0.317018838765051,0.333333333333333,0.317018838765051,0.333333333333333),
(1.,0.951056516295154,1.,0.951056516295154,1.,0.951056516295154,1.,0.951056516295154,
1.,0.951056516295154,1.,0.951056516295154,1.,0.951056516295154,1.,0.951056516295154,
1.,0.951056516295154,1.,0.951056516295154,1.,0.951056516295154,1.,0.951056516295154,
1.,0.951056516295154,1.,0.951056516295154,1.,0.951056516295154,1.,0.951056516295154,
1.,0.951056516295154,1.,0.951056516295154,1.,0.951056516295154,1.,0.951056516295154,
1.,0.951056516295154,1.,0.951056516295154,1.,0.951056516295154,1.,0.951056516295154,
1.,0.951056516295154,1.,0.951056516295154,1.,0.951056516295154,1.,0.951056516295154,
1.,0.951056516295154,1.,0.951056516295154,1.,0.951056516295154,1.,0.951056516295154,
1.,0.951056516295154,1.,0.951056516295154,1.,0.951056516295154,1.,0.951056516295154,
1.,0.951056516295154,1.,0.951056516295154,1.,0.951056516295154,1.,0.951056516295154,
1.,0.951056516295154,1.,0.951056516295154,1.,0.951056516295154,1.,0.951056516295154,
1.,0.951056516295154,1.,0.951056516295154,1.,0.951056516295154,1.,0.951056516295154,
1.,0.951056516295154,1.,0.951056516295154,1.,0.951056516295154,1.,0.951056516295154,
1.,0.951056516295154,1.,0.951056516295154,1.,0.951056516295154,1.,0.951056516295154,
1.,0.951056516295154,1.,0.951056516295154,1.,0.951056516295154,1.,0.951056516295154,
1.,0.951056516295154,1.,0.951056516295154,1.,0.951056516295154,1.,0.951056516295154,
1.,0.951056516295154,1.,0.951056516295154,1.,0.951056516295154,1.,0.951056516295154,
1.,0.951056516295154,1.,0.951056516295154,1.,0.951056516295154,1.,0.951056516295154,
1.,0.951056516295154,1.,0.951056516295154,1.,0.951056516295154,1.,0.951056516295154,
1.,0.951056516295154,1.,0.951056516295154,1.,0.951056516295154,1.,0.951056516295154,
1.,0.951056516295154,1.,0.951056516295154,1.,0.951056516295154,1.,0.951056516295154,
1.,0.951056516295154,1.,0.951056516295154,1.,0.951056516295154,1.,0.951056516295154,
1.,0.951056516295154,1.,0.951056516295154,1.,0.951056516295154,1.,0.951056516295154,
1.,0.951056516295154,1.,0.951056516295154,1.,0.951056516295154,1.,0.951056516295154,
1.,0.951056516295154,1.,0.951056516295154,1.,0.951056516295154,1.,0.951056516295154,
1.),(0.333333333333333,0.317018838765051,0.333333333333333,0.317018838765051,
0.333333333333333,0.317018838765051,0.333333333333333,0.317018838765051,
0.333333333333333,0.317018838765051,0.333333333333333,0.317018838765051,
0.333333333333333,0.317018838765051,0.333333333333333,0.317018838765051,
0.333333333333333,0.317018838765051,0.333333333333333,0.317018838765051,
0.333333333333333,0.317018838765051,0.333333333333333,0.317018838765051,
0.333333333333333,0.317018838765051,0.333333333333333,0.317018838765051,
0.333333333333333,0.317018838765051,0.333333333333333,0.317018838765051,
0.333333333333333,0.317018838765051,0.333333333333333,0.317018838765051,
0.333333333333333,0.317018838765051,0.333333333333333,0.317018838765051,
0.333333333333333,0.317018838765051,0.333333333333333,0.317018838765051,
0.333333333333333,0.317018838765051,0.333333333333333,0.317018838765051,
0.333333333333333,0.317018838765051,0.333333333333333,0.317018838765051,
0.333333333333333,0.317018838765051,0.333333333333333,0.317018838765051,
0.333333333333333,0.317018838765051,0.333333333333333,0.317018838765051,
0.333333333333333,0.317018838765051,0.333333333333333,0.317018838765051,
0.333333333333333,0.317018838765051,0.333333333333333,0.317018838765051,
0.333333333333333,0.317018838765051,0.333333333333333,0.317018838765051,
0.333333333333333,0.317018838765051,0.333333333333333,0.317018838765051,
0.333333333333333,0.317018838765051,0.333333333333333,0.317018838765051,
0.333333333333333,0.317018838765051,0.333333333333333,0.317018838765051,
0.333333333333333,0.317018838765051,0.333333333333333,0.317018838765051,
0.333333333333333,0.317018838765051,0.333333333333333,0.317018838765051,
0.333333333333333,0.317018838765051,0.333333333333333,0.317018838765051,
0.333333333333333,0.317018838765051,0.333333333333333,0.317018838765051,
0.333333333333333,0.317018838765051,0.333333333333333,0.317018838765051,
0.333333333333333,0.317018838765051,0.333333333333333,0.317018838765051,
0.333333333333333,0.317018838765051,0.333333333333333,0.317018838765051,
0.333333333333333,0.317018838765051,0.333333333333333,0.317018838765051,
0.333333333333333,0.317018838765051,0.333333333333333,0.317018838765051,
0.333333333333333,0.317018838765051,0.333333333333333,0.317018838765051,
0.333333333333333,0.317018838765051,0.333333333333333,0.317018838765051,
0.333333333333333,0.317018838765051,0.333333333333333,0.317018838765051,
0.333333333333333,0.317018838765051,0.333333333333333,0.317018838765051,
0.333333333333333,0.317018838765051,0.333333333333333,0.317018838765051,
0.333333333333333,0.317018838765051,0.333333333333333,0.317018838765051,
0.333333333333333,0.317018838765051,0.333333333333333,0.317018838765051,
0.333333333333333,0.317018838765051,0.333333333333333,0.317018838765051,
0.333333333333333,0.317018838765051,0.333333333333333,0.317018838765051,
0.333333333333333,0.317018838765051,0.333333333333333,0.317018838765051,
0.333333333333333,0.317018838765051,0.333333333333333,0.317018838765051,
0.333333333333333,0.317018838765051,0.333333333333333,0.317018838765051,
0.333333333333333,0.317018838765051,0.333333333333333,0.317018838765051,
0.333333333333333,0.317018838765051,0.333333333333333,0.317018838765051,
0.333333333333333,0.317018838765051,0.333333333333333,0.317018838765051,
0.333333333333333,0.317018838765051,0.333333333333333,0.317018838765051,
0.333333333333333,0.317018838765051,0.333333333333333,0.317018838765051,
0.333333333333333,0.317018838765051,0.333333333333333,0.317018838765051,
0.333333333333333,0.317018838765051,0.333333333333333,0.317018838765051,
0.333333333333333,0.317018838765051,0.333333333333333,0.317018838765051,
0.333333333333333),(0.333333333333333,0.317018838765051,0.333333333333333,
0.317018838765051,0.333333333333333,0.317018838765051,0.333333333333333,
0.317018838765051,0.333333333333333,0.317018838765051,0.333333333333333,
0.317018838765051,0.333333333333333,0.317018838765051,0.333333333333333,
0.317018838765051,0.333333333333333,0.317018838765051,0.333333333333333,
0.317018838765051,0.333333333333333,0.317018838765051,0.333333333333333,
0.317018838765051,0.333333333333333,0.317018838765051,0.333333333333333,
0.317018838765051,0.333333333333333,0.317018838765051,0.333333333333333,
0.317018838765051,0.333333333333333,0.317018838765051,0.333333333333333,
0.317018838765051,0.333333333333333,0.317018838765051,0.333333333333333,
0.317018838765051,0.333333333333333,0.317018838765051,0.333333333333333,
0.317018838765051,0.333333333333333,0.317018838765051,0.333333333333333,
0.317018838765051,0.333333333333333,0.317018838765051,0.333333333333333,
0.317018838765051,0.333333333333333,0.317018838765051,0.333333333333333,
0.317018838765051,0.333333333333333,0.317018838765051,0.333333333333333,
0.317018838765051,0.333333333333333,0.317018838765051,0.333333333333333,
0.317018838765051,0.333333333333333,0.317018838765051,0.333333333333333,
0.317018838765051,0.333333333333333,0.317018838765051,0.333333333333333,
0.317018838765051,0.333333333333333,0.317018838765051,0.333333333333333,
0.317018838765051,0.333333333333333,0.317018838765051,0.333333333333333,
0.317018838765051,0.333333333333333,0.317018838765051,0.333333333333333,
0.317018838765051,0.333333333333333,0.317018838765051,0.333333333333333,
0.317018838765051,0.333333333333333,0.317018838765051,0.333333333333333,
0.317018838765051,0.333333333333333,0.317018838765051,0.333333333333333,
0.317018838765051,0.333333333333333,0.317018838765051,0.333333333333333,
0.317018838765051,0.333333333333333,0.317018838765051,0.333333333333333,
0.317018838765051,0.333333333333333,0.317018838765051,0.333333333333333,
0.317018838765051,0.333333333333333,0.317018838765051,0.333333333333333,
0.317018838765051,0.333333333333333,0.317018838765051,0.333333333333333,
0.317018838765051,0.333333333333333,0.317018838765051,0.333333333333333,
0.317018838765051,0.333333333333333,0.317018838765051,0.333333333333333,
0.317018838765051,0.333333333333333,0.317018838765051,0.333333333333333,
0.317018838765051,0.333333333333333,0.317018838765051,0.333333333333333,
0.317018838765051,0.333333333333333,0.317018838765051,0.333333333333333,
0.317018838765051,0.333333333333333,0.317018838765051,0.333333333333333,
0.317018838765051,0.333333333333333,0.317018838765051,0.333333333333333,
0.317018838765051,0.333333333333333,0.317018838765051,0.333333333333333,
0.317018838765051,0.333333333333333,0.317018838765051,0.333333333333333,
0.317018838765051,0.333333333333333,0.317018838765051,0.333333333333333,
0.317018838765051,0.333333333333333,0.317018838765051,0.333333333333333,
0.317018838765051,0.333333333333333,0.317018838765051,0.333333333333333,
0.317018838765051,0.333333333333333,0.317018838765051,0.333333333333333,
0.317018838765051,0.333333333333333,0.317018838765051,0.333333333333333,
0.317018838765051,0.333333333333333,0.317018838765051,0.333333333333333,
0.317018838765051,0.333333333333333,0.317018838765051,0.333333333333333,
0.317018838765051,0.333333333333333,0.317018838765051,0.333333333333333,
0.317018838765051,0.333333333333333,0.317018838765051,0.333333333333333,
0.317018838765051,0.333333333333333,0.317018838765051,0.333333333333333,
0.317018838765051,0.333333333333333,0.317018838765051,0.333333333333333,
0.317018838765051,0.333333333333333,0.317018838765051,0.333333333333333,
0.317018838765051,0.333333333333333),(1.,0.951056516295154,1.,0.951056516295154,
1.,0.951056516295154,1.,0.951056516295154,1.,0.951056516295154,1.,0.951056516295154,
1.,0.951056516295154,1.,0.951056516295154,1.,0.951056516295154,1.,0.951056516295154,
1.,0.951056516295154,1.,0.951056516295154,1.,0.951056516295154,1.,0.951056516295154,
1.,0.951056516295154,1.,0.951056516295154,1.,0.951056516295154,1.,0.951056516295154,
1.,0.951056516295154,1.,0.951056516295154,1.,0.951056516295154,1.,0.951056516295154,
1.,0.951056516295154,1.,0.951056516295154,1.,0.951056516295154,1.,0.951056516295154,
1.,0.951056516295154,1.,0.951056516295154,1.,0.951056516295154,1.,0.951056516295154,
1.,0.951056516295154,1.,0.951056516295154,1.,0.951056516295154,1.,0.951056516295154,
1.,0.951056516295154,1.,0.951056516295154,1.,0.951056516295154,1.,0.951056516295154,
1.,0.951056516295154,1.,0.951056516295154,1.,0.951056516295154,1.,0.951056516295154,
1.,0.951056516295154,1.,0.951056516295154,1.,0.951056516295154,1.,0.951056516295154,
1.,0.951056516295154,1.,0.951056516295154,1.,0.951056516295154,1.,0.951056516295154,
1.,0.951056516295154,1.,0.951056516295154,1.,0.951056516295154,1.,0.951056516295154,
1.,0.951056516295154,1.,0.951056516295154,1.,0.951056516295154,1.,0.951056516295154,
1.,0.951056516295154,1.,0.951056516295154,1.,0.951056516295154,1.,0.951056516295154,
1.,0.951056516295154,1.,0.951056516295154,1.,0.951056516295154,1.,0.951056516295154,
1.,0.951056516295154,1.,0.951056516295154,1.,0.951056516295154,1.,0.951056516295154,
1.,0.951056516295154,1.,0.951056516295154,1.,0.951056516295154,1.,0.951056516295154,
1.,0.951056516295154,1.,0.951056516295154,1.,0.951056516295154,1.,0.951056516295154,
1.,0.951056516295154,1.,0.951056516295154,1.,0.951056516295154,1.,0.951056516295154,
1.,0.951056516295154,1.,0.951056516295154,1.,0.951056516295154,1.,0.951056516295154,
1.,0.951056516295154,1.,0.951056516295154,1.,0.951056516295154,1.,0.951056516295154,
1.,0.951056516295154,1.,0.951056516295154,1.,0.951056516295154,1.,0.951056516295154,
1.,0.951056516295154,1.,0.951056516295154,1.,0.951056516295154,1.,0.951056516295154,
1.,0.951056516295154,1.,0.951056516295154,1.)))
REPRESENTATION_ITEM('')
SURFACE()
);
#96=(
BOUNDED_SURFACE()
B_SPLINE_SURFACE(3,2,((#5662,#5663,#5664,#5665,#5666,#5667,#5668,#5669,
#5670,#5671,#5672,#5673,#5674,#5675,#5676,#5677,#5678,#5679,#5680,#5681,
#5682,#5683,#5684,#5685,#5686,#5687,#5688,#5689,#5690,#5691,#5692,#5693,
#5694,#5695,#5696,#5697,#5698,#5699,#5700,#5701,#5702,#5703,#5704,#5705,
#5706,#5707,#5708,#5709,#5710,#5711,#5712,#5713,#5714,#5715,#5716,#5717,
#5718,#5719,#5720,#5721,#5722,#5723,#5724,#5725,#5726,#5727,#5728,#5729,
#5730,#5731,#5732,#5733,#5734,#5735,#5736,#5737,#5738,#5739,#5740,#5741,
#5742,#5743,#5744,#5745,#5746,#5747,#5748,#5749,#5750,#5751,#5752,#5753,
#5754,#5755,#5756,#5757,#5758,#5759,#5760,#5761,#5762,#5763,#5764,#5765,
#5766,#5767,#5768,#5769,#5770,#5771,#5772,#5773,#5774,#5775,#5776,#5777,
#5778,#5779,#5780,#5781,#5782,#5783,#5784,#5785,#5786,#5787,#5788,#5789,
#5790,#5791,#5792,#5793,#5794,#5795,#5796,#5797,#5798,#5799,#5800,#5801,
#5802,#5803,#5804,#5805,#5806,#5807,#5808,#5809,#5810,#5811,#5812,#5813,
#5814,#5815,#5816,#5817,#5818,#5819,#5820,#5821,#5822,#5823,#5824,#5825,
#5826,#5827,#5828,#5829,#5830,#5831,#5832,#5833,#5834,#5835,#5836,#5837,
#5838,#5839,#5840,#5841,#5842,#5843,#5844,#5845,#5846,#5847,#5848,#5849,
#5850,#5851,#5852,#5853,#5854,#5855,#5856,#5857,#5858,#5859,#5860,#5861,
#5862),(#5863,#5864,#5865,#5866,#5867,#5868,#5869,#5870,#5871,#5872,#5873,
#5874,#5875,#5876,#5877,#5878,#5879,#5880,#5881,#5882,#5883,#5884,#5885,
#5886,#5887,#5888,#5889,#5890,#5891,#5892,#5893,#5894,#5895,#5896,#5897,
#5898,#5899,#5900,#5901,#5902,#5903,#5904,#5905,#5906,#5907,#5908,#5909,
#5910,#5911,#5912,#5913,#5914,#5915,#5916,#5917,#5918,#5919,#5920,#5921,
#5922,#5923,#5924,#5925,#5926,#5927,#5928,#5929,#5930,#5931,#5932,#5933,
#5934,#5935,#5936,#5937,#5938,#5939,#5940,#5941,#5942,#5943,#5944,#5945,
#5946,#5947,#5948,#5949,#5950,#5951,#5952,#5953,#5954,#5955,#5956,#5957,
#5958,#5959,#5960,#5961,#5962,#5963,#5964,#5965,#5966,#5967,#5968,#5969,
#5970,#5971,#5972,#5973,#5974,#5975,#5976,#5977,#5978,#5979,#5980,#5981,
#5982,#5983,#5984,#5985,#5986,#5987,#5988,#5989,#5990,#5991,#5992,#5993,
#5994,#5995,#5996,#5997,#5998,#5999,#6000,#6001,#6002,#6003,#6004,#6005,
#6006,#6007,#6008,#6009,#6010,#6011,#6012,#6013,#6014,#6015,#6016,#6017,
#6018,#6019,#6020,#6021,#6022,#6023,#6024,#6025,#6026,#6027,#6028,#6029,
#6030,#6031,#6032,#6033,#6034,#6035,#6036,#6037,#6038,#6039,#6040,#6041,
#6042,#6043,#6044,#6045,#6046,#6047,#6048,#6049,#6050,#6051,#6052,#6053,
#6054,#6055,#6056,#6057,#6058,#6059,#6060,#6061,#6062,#6063),(#6064,#6065,
#6066,#6067,#6068,#6069,#6070,#6071,#6072,#6073,#6074,#6075,#6076,#6077,
#6078,#6079,#6080,#6081,#6082,#6083,#6084,#6085,#6086,#6087,#6088,#6089,
#6090,#6091,#6092,#6093,#6094,#6095,#6096,#6097,#6098,#6099,#6100,#6101,
#6102,#6103,#6104,#6105,#6106,#6107,#6108,#6109,#6110,#6111,#6112,#6113,
#6114,#6115,#6116,#6117,#6118,#6119,#6120,#6121,#6122,#6123,#6124,#6125,
#6126,#6127,#6128,#6129,#6130,#6131,#6132,#6133,#6134,#6135,#6136,#6137,
#6138,#6139,#6140,#6141,#6142,#6143,#6144,#6145,#6146,#6147,#6148,#6149,
#6150,#6151,#6152,#6153,#6154,#6155,#6156,#6157,#6158,#6159,#6160,#6161,
#6162,#6163,#6164,#6165,#6166,#6167,#6168,#6169,#6170,#6171,#6172,#6173,
#6174,#6175,#6176,#6177,#6178,#6179,#6180,#6181,#6182,#6183,#6184,#6185,
#6186,#6187,#6188,#6189,#6190,#6191,#6192,#6193,#6194,#6195,#6196,#6197,
#6198,#6199,#6200,#6201,#6202,#6203,#6204,#6205,#6206,#6207,#6208,#6209,
#6210,#6211,#6212,#6213,#6214,#6215,#6216,#6217,#6218,#6219,#6220,#6221,
#6222,#6223,#6224,#6225,#6226,#6227,#6228,#6229,#6230,#6231,#6232,#6233,
#6234,#6235,#6236,#6237,#6238,#6239,#6240,#6241,#6242,#6243,#6244,#6245,
#6246,#6247,#6248,#6249,#6250,#6251,#6252,#6253,#6254,#6255,#6256,#6257,
#6258,#6259,#6260,#6261,#6262,#6263,#6264),(#6265,#6266,#6267,#6268,#6269,
#6270,#6271,#6272,#6273,#6274,#6275,#6276,#6277,#6278,#6279,#6280,#6281,
#6282,#6283,#6284,#6285,#6286,#6287,#6288,#6289,#6290,#6291,#6292,#6293,
#6294,#6295,#6296,#6297,#6298,#6299,#6300,#6301,#6302,#6303,#6304,#6305,
#6306,#6307,#6308,#6309,#6310,#6311,#6312,#6313,#6314,#6315,#6316,#6317,
#6318,#6319,#6320,#6321,#6322,#6323,#6324,#6325,#6326,#6327,#6328,#6329,
#6330,#6331,#6332,#6333,#6334,#6335,#6336,#6337,#6338,#6339,#6340,#6341,
#6342,#6343,#6344,#6345,#6346,#6347,#6348,#6349,#6350,#6351,#6352,#6353,
#6354,#6355,#6356,#6357,#6358,#6359,#6360,#6361,#6362,#6363,#6364,#6365,
#6366,#6367,#6368,#6369,#6370,#6371,#6372,#6373,#6374,#6375,#6376,#6377,
#6378,#6379,#6380,#6381,#6382,#6383,#6384,#6385,#6386,#6387,#6388,#6389,
#6390,#6391,#6392,#6393,#6394,#6395,#6396,#6397,#6398,#6399,#6400,#6401,
#6402,#6403,#6404,#6405,#6406,#6407,#6408,#6409,#6410,#6411,#6412,#6413,
#6414,#6415,#6416,#6417,#6418,#6419,#6420,#6421,#6422,#6423,#6424,#6425,
#6426,#6427,#6428,#6429,#6430,#6431,#6432,#6433,#6434,#6435,#6436,#6437,
#6438,#6439,#6440,#6441,#6442,#6443,#6444,#6445,#6446,#6447,#6448,#6449,
#6450,#6451,#6452,#6453,#6454,#6455,#6456,#6457,#6458,#6459,#6460,#6461,
#6462,#6463,#6464,#6465),(#6466,#6467,#6468,#6469,#6470,#6471,#6472,#6473,
#6474,#6475,#6476,#6477,#6478,#6479,#6480,#6481,#6482,#6483,#6484,#6485,
#6486,#6487,#6488,#6489,#6490,#6491,#6492,#6493,#6494,#6495,#6496,#6497,
#6498,#6499,#6500,#6501,#6502,#6503,#6504,#6505,#6506,#6507,#6508,#6509,
#6510,#6511,#6512,#6513,#6514,#6515,#6516,#6517,#6518,#6519,#6520,#6521,
#6522,#6523,#6524,#6525,#6526,#6527,#6528,#6529,#6530,#6531,#6532,#6533,
#6534,#6535,#6536,#6537,#6538,#6539,#6540,#6541,#6542,#6543,#6544,#6545,
#6546,#6547,#6548,#6549,#6550,#6551,#6552,#6553,#6554,#6555,#6556,#6557,
#6558,#6559,#6560,#6561,#6562,#6563,#6564,#6565,#6566,#6567,#6568,#6569,
#6570,#6571,#6572,#6573,#6574,#6575,#6576,#6577,#6578,#6579,#6580,#6581,
#6582,#6583,#6584,#6585,#6586,#6587,#6588,#6589,#6590,#6591,#6592,#6593,
#6594,#6595,#6596,#6597,#6598,#6599,#6600,#6601,#6602,#6603,#6604,#6605,
#6606,#6607,#6608,#6609,#6610,#6611,#6612,#6613,#6614,#6615,#6616,#6617,
#6618,#6619,#6620,#6621,#6622,#6623,#6624,#6625,#6626,#6627,#6628,#6629,
#6630,#6631,#6632,#6633,#6634,#6635,#6636,#6637,#6638,#6639,#6640,#6641,
#6642,#6643,#6644,#6645,#6646,#6647,#6648,#6649,#6650,#6651,#6652,#6653,
#6654,#6655,#6656,#6657,#6658,#6659,#6660,#6661,#6662,#6663,#6664,#6665,
#6666),(#6667,#6668,#6669,#6670,#6671,#6672,#6673,#6674,#6675,#6676,#6677,
#6678,#6679,#6680,#6681,#6682,#6683,#6684,#6685,#6686,#6687,#6688,#6689,
#6690,#6691,#6692,#6693,#6694,#6695,#6696,#6697,#6698,#6699,#6700,#6701,
#6702,#6703,#6704,#6705,#6706,#6707,#6708,#6709,#6710,#6711,#6712,#6713,
#6714,#6715,#6716,#6717,#6718,#6719,#6720,#6721,#6722,#6723,#6724,#6725,
#6726,#6727,#6728,#6729,#6730,#6731,#6732,#6733,#6734,#6735,#6736,#6737,
#6738,#6739,#6740,#6741,#6742,#6743,#6744,#6745,#6746,#6747,#6748,#6749,
#6750,#6751,#6752,#6753,#6754,#6755,#6756,#6757,#6758,#6759,#6760,#6761,
#6762,#6763,#6764,#6765,#6766,#6767,#6768,#6769,#6770,#6771,#6772,#6773,
#6774,#6775,#6776,#6777,#6778,#6779,#6780,#6781,#6782,#6783,#6784,#6785,
#6786,#6787,#6788,#6789,#6790,#6791,#6792,#6793,#6794,#6795,#6796,#6797,
#6798,#6799,#6800,#6801,#6802,#6803,#6804,#6805,#6806,#6807,#6808,#6809,
#6810,#6811,#6812,#6813,#6814,#6815,#6816,#6817,#6818,#6819,#6820,#6821,
#6822,#6823,#6824,#6825,#6826,#6827,#6828,#6829,#6830,#6831,#6832,#6833,
#6834,#6835,#6836,#6837,#6838,#6839,#6840,#6841,#6842,#6843,#6844,#6845,
#6846,#6847,#6848,#6849,#6850,#6851,#6852,#6853,#6854,#6855,#6856,#6857,
#6858,#6859,#6860,#6861,#6862,#6863,#6864,#6865,#6866,#6867),(#6868,#6869,
#6870,#6871,#6872,#6873,#6874,#6875,#6876,#6877,#6878,#6879,#6880,#6881,
#6882,#6883,#6884,#6885,#6886,#6887,#6888,#6889,#6890,#6891,#6892,#6893,
#6894,#6895,#6896,#6897,#6898,#6899,#6900,#6901,#6902,#6903,#6904,#6905,
#6906,#6907,#6908,#6909,#6910,#6911,#6912,#6913,#6914,#6915,#6916,#6917,
#6918,#6919,#6920,#6921,#6922,#6923,#6924,#6925,#6926,#6927,#6928,#6929,
#6930,#6931,#6932,#6933,#6934,#6935,#6936,#6937,#6938,#6939,#6940,#6941,
#6942,#6943,#6944,#6945,#6946,#6947,#6948,#6949,#6950,#6951,#6952,#6953,
#6954,#6955,#6956,#6957,#6958,#6959,#6960,#6961,#6962,#6963,#6964,#6965,
#6966,#6967,#6968,#6969,#6970,#6971,#6972,#6973,#6974,#6975,#6976,#6977,
#6978,#6979,#6980,#6981,#6982,#6983,#6984,#6985,#6986,#6987,#6988,#6989,
#6990,#6991,#6992,#6993,#6994,#6995,#6996,#6997,#6998,#6999,#7000,#7001,
#7002,#7003,#7004,#7005,#7006,#7007,#7008,#7009,#7010,#7011,#7012,#7013,
#7014,#7015,#7016,#7017,#7018,#7019,#7020,#7021,#7022,#7023,#7024,#7025,
#7026,#7027,#7028,#7029,#7030,#7031,#7032,#7033,#7034,#7035,#7036,#7037,
#7038,#7039,#7040,#7041,#7042,#7043,#7044,#7045,#7046,#7047,#7048,#7049,
#7050,#7051,#7052,#7053,#7054,#7055,#7056,#7057,#7058,#7059,#7060,#7061,
#7062,#7063,#7064,#7065,#7066,#7067,#7068)),.UNSPECIFIED.,.T.,.F.,.F.)
B_SPLINE_SURFACE_WITH_KNOTS((4,3,4),(3,2,2,2,2,2,2,2,2,2,2,2,2,2,2,2,2,
2,2,2,2,2,2,2,2,2,2,2,2,2,2,2,2,2,2,2,2,2,2,2,2,2,2,2,2,2,2,2,2,2,2,2,2,
2,2,2,2,2,2,2,2,2,2,2,2,2,2,2,2,2,2,2,2,2,2,2,2,2,2,2,2,2,2,2,2,2,2,2,2,
2,2,2,2,2,2,2,2,2,2,2,3),(0.,0.5,1.),(0.,0.01,0.02,0.03,0.04,0.05,0.06,
0.07,0.08,0.09,0.1,0.11,0.12,0.13,0.14,0.15,0.16,0.17,0.18,0.19,0.2,0.21,
0.22,0.23,0.24,0.25,0.26,0.27,0.28,0.29,0.3,0.31,0.32,0.33,0.34,0.35,0.36,
0.37,0.38,0.39,0.4,0.41,0.42,0.43,0.44,0.45,0.46,0.47,0.48,0.49,0.5,0.51,
0.52,0.53,0.54,0.55,0.56,0.57,0.58,0.59,0.6,0.61,0.62,0.63,0.64,0.65,0.66,
0.67,0.68,0.69,0.7,0.71,0.72,0.73,0.74,0.75,0.76,0.77,0.78,0.79,0.8,0.81,
0.82,0.83,0.84,0.85,0.86,0.87,0.88,0.89,0.9,0.91,0.92,0.93,0.94,0.95,0.96,
0.97,0.98,0.99,1.),.UNSPECIFIED.)
GEOMETRIC_REPRESENTATION_ITEM()
RATIONAL_B_SPLINE_SURFACE(((1.,0.951056516295154,1.,0.951056516295154,1.,
0.951056516295154,1.,0.951056516295154,1.,0.951056516295154,1.,0.951056516295154,
1.,0.951056516295154,1.,0.951056516295154,1.,0.951056516295154,1.,0.951056516295154,
1.,0.951056516295154,1.,0.951056516295154,1.,0.951056516295154,1.,0.951056516295154,
1.,0.951056516295154,1.,0.951056516295154,1.,0.951056516295154,1.,0.951056516295154,
1.,0.951056516295154,1.,0.951056516295154,1.,0.951056516295154,1.,0.951056516295154,
1.,0.951056516295154,1.,0.951056516295154,1.,0.951056516295154,1.,0.951056516295154,
1.,0.951056516295154,1.,0.951056516295154,1.,0.951056516295154,1.,0.951056516295154,
1.,0.951056516295154,1.,0.951056516295154,1.,0.951056516295154,1.,0.951056516295154,
1.,0.951056516295154,1.,0.951056516295154,1.,0.951056516295154,1.,0.951056516295154,
1.,0.951056516295154,1.,0.951056516295154,1.,0.951056516295154,1.,0.951056516295154,
1.,0.951056516295154,1.,0.951056516295154,1.,0.951056516295154,1.,0.951056516295154,
1.,0.951056516295154,1.,0.951056516295154,1.,0.951056516295154,1.,0.951056516295154,
1.,0.951056516295154,1.,0.951056516295154,1.,0.951056516295154,1.,0.951056516295154,
1.,0.951056516295154,1.,0.951056516295154,1.,0.951056516295154,1.,0.951056516295154,
1.,0.951056516295154,1.,0.951056516295154,1.,0.951056516295154,1.,0.951056516295154,
1.,0.951056516295154,1.,0.951056516295154,1.,0.951056516295154,1.,0.951056516295154,
1.,0.951056516295154,1.,0.951056516295154,1.,0.951056516295154,1.,0.951056516295154,
1.,0.951056516295154,1.,0.951056516295154,1.,0.951056516295154,1.,0.951056516295154,
1.,0.951056516295154,1.,0.951056516295154,1.,0.951056516295154,1.,0.951056516295154,
1.,0.951056516295154,1.,0.951056516295154,1.,0.951056516295154,1.,0.951056516295154,
1.,0.951056516295154,1.,0.951056516295154,1.,0.951056516295154,1.,0.951056516295154,
1.,0.951056516295154,1.,0.951056516295154,1.,0.951056516295154,1.,0.951056516295154,
1.,0.951056516295154,1.,0.951056516295154,1.,0.951056516295154,1.,0.951056516295154,
1.,0.951056516295154,1.,0.951056516295154,1.,0.951056516295154,1.,0.951056516295154,
1.,0.951056516295154,1.,0.951056516295154,1.),(0.333333333333333,0.317018838765051,
0.333333333333333,0.317018838765051,0.333333333333333,0.317018838765051,
0.333333333333333,0.317018838765051,0.333333333333333,0.317018838765051,
0.333333333333333,0.317018838765051,0.333333333333333,0.317018838765051,
0.333333333333333,0.317018838765051,0.333333333333333,0.317018838765051,
0.333333333333333,0.317018838765051,0.333333333333333,0.317018838765051,
0.333333333333333,0.317018838765051,0.333333333333333,0.317018838765051,
0.333333333333333,0.317018838765051,0.333333333333333,0.317018838765051,
0.333333333333333,0.317018838765051,0.333333333333333,0.317018838765051,
0.333333333333333,0.317018838765051,0.333333333333333,0.317018838765051,
0.333333333333333,0.317018838765051,0.333333333333333,0.317018838765051,
0.333333333333333,0.317018838765051,0.333333333333333,0.317018838765051,
0.333333333333333,0.317018838765051,0.333333333333333,0.317018838765051,
0.333333333333333,0.317018838765051,0.333333333333333,0.317018838765051,
0.333333333333333,0.317018838765051,0.333333333333333,0.317018838765051,
0.333333333333333,0.317018838765051,0.333333333333333,0.317018838765051,
0.333333333333333,0.317018838765051,0.333333333333333,0.317018838765051,
0.333333333333333,0.317018838765051,0.333333333333333,0.317018838765051,
0.333333333333333,0.317018838765051,0.333333333333333,0.317018838765051,
0.333333333333333,0.317018838765051,0.333333333333333,0.317018838765051,
0.333333333333333,0.317018838765051,0.333333333333333,0.317018838765051,
0.333333333333333,0.317018838765051,0.333333333333333,0.317018838765051,
0.333333333333333,0.317018838765051,0.333333333333333,0.317018838765051,
0.333333333333333,0.317018838765051,0.333333333333333,0.317018838765051,
0.333333333333333,0.317018838765051,0.333333333333333,0.317018838765051,
0.333333333333333,0.317018838765051,0.333333333333333,0.317018838765051,
0.333333333333333,0.317018838765051,0.333333333333333,0.317018838765051,
0.333333333333333,0.317018838765051,0.333333333333333,0.317018838765051,
0.333333333333333,0.317018838765051,0.333333333333333,0.317018838765051,
0.333333333333333,0.317018838765051,0.333333333333333,0.317018838765051,
0.333333333333333,0.317018838765051,0.333333333333333,0.317018838765051,
0.333333333333333,0.317018838765051,0.333333333333333,0.317018838765051,
0.333333333333333,0.317018838765051,0.333333333333333,0.317018838765051,
0.333333333333333,0.317018838765051,0.333333333333333,0.317018838765051,
0.333333333333333,0.317018838765051,0.333333333333333,0.317018838765051,
0.333333333333333,0.317018838765051,0.333333333333333,0.317018838765051,
0.333333333333333,0.317018838765051,0.333333333333333,0.317018838765051,
0.333333333333333,0.317018838765051,0.333333333333333,0.317018838765051,
0.333333333333333,0.317018838765051,0.333333333333333,0.317018838765051,
0.333333333333333,0.317018838765051,0.333333333333333,0.317018838765051,
0.333333333333333,0.317018838765051,0.333333333333333,0.317018838765051,
0.333333333333333,0.317018838765051,0.333333333333333,0.317018838765051,
0.333333333333333,0.317018838765051,0.333333333333333,0.317018838765051,
0.333333333333333,0.317018838765051,0.333333333333333,0.317018838765051,
0.333333333333333,0.317018838765051,0.333333333333333,0.317018838765051,
0.333333333333333,0.317018838765051,0.333333333333333,0.317018838765051,
0.333333333333333,0.317018838765051,0.333333333333333,0.317018838765051,
0.333333333333333,0.317018838765051,0.333333333333333,0.317018838765051,
0.333333333333333,0.317018838765051,0.333333333333333,0.317018838765051,
0.333333333333333,0.317018838765051,0.333333333333333,0.317018838765051,
0.333333333333333,0.317018838765051,0.333333333333333),(0.333333333333333,
0.317018838765051,0.333333333333333,0.317018838765051,0.333333333333333,
0.317018838765051,0.333333333333333,0.317018838765051,0.333333333333333,
0.317018838765051,0.333333333333333,0.317018838765051,0.333333333333333,
0.317018838765051,0.333333333333333,0.317018838765051,0.333333333333333,
0.317018838765051,0.333333333333333,0.317018838765051,0.333333333333333,
0.317018838765051,0.333333333333333,0.317018838765051,0.333333333333333,
0.317018838765051,0.333333333333333,0.317018838765051,0.333333333333333,
0.317018838765051,0.333333333333333,0.317018838765051,0.333333333333333,
0.317018838765051,0.333333333333333,0.317018838765051,0.333333333333333,
0.317018838765051,0.333333333333333,0.317018838765051,0.333333333333333,
0.317018838765051,0.333333333333333,0.317018838765051,0.333333333333333,
0.317018838765051,0.333333333333333,0.317018838765051,0.333333333333333,
0.317018838765051,0.333333333333333,0.317018838765051,0.333333333333333,
0.317018838765051,0.333333333333333,0.317018838765051,0.333333333333333,
0.317018838765051,0.333333333333333,0.317018838765051,0.333333333333333,
0.317018838765051,0.333333333333333,0.317018838765051,0.333333333333333,
0.317018838765051,0.333333333333333,0.317018838765051,0.333333333333333,
0.317018838765051,0.333333333333333,0.317018838765051,0.333333333333333,
0.317018838765051,0.333333333333333,0.317018838765051,0.333333333333333,
0.317018838765051,0.333333333333333,0.317018838765051,0.333333333333333,
0.317018838765051,0.333333333333333,0.317018838765051,0.333333333333333,
0.317018838765051,0.333333333333333,0.317018838765051,0.333333333333333,
0.317018838765051,0.333333333333333,0.317018838765051,0.333333333333333,
0.317018838765051,0.333333333333333,0.317018838765051,0.333333333333333,
0.317018838765051,0.333333333333333,0.317018838765051,0.333333333333333,
0.317018838765051,0.333333333333333,0.317018838765051,0.333333333333333,
0.317018838765051,0.333333333333333,0.317018838765051,0.333333333333333,
0.317018838765051,0.333333333333333,0.317018838765051,0.333333333333333,
0.317018838765051,0.333333333333333,0.317018838765051,0.333333333333333,
0.317018838765051,0.333333333333333,0.317018838765051,0.333333333333333,
0.317018838765051,0.333333333333333,0.317018838765051,0.333333333333333,
0.317018838765051,0.333333333333333,0.317018838765051,0.333333333333333,
0.317018838765051,0.333333333333333,0.317018838765051,0.333333333333333,
0.317018838765051,0.333333333333333,0.317018838765051,0.333333333333333,
0.317018838765051,0.333333333333333,0.317018838765051,0.333333333333333,
0.317018838765051,0.333333333333333,0.317018838765051,0.333333333333333,
0.317018838765051,0.333333333333333,0.317018838765051,0.333333333333333,
0.317018838765051,0.333333333333333,0.317018838765051,0.333333333333333,
0.317018838765051,0.333333333333333,0.317018838765051,0.333333333333333,
0.317018838765051,0.333333333333333,0.317018838765051,0.333333333333333,
0.317018838765051,0.333333333333333,0.317018838765051,0.333333333333333,
0.317018838765051,0.333333333333333,0.317018838765051,0.333333333333333,
0.317018838765051,0.333333333333333,0.317018838765051,0.333333333333333,
0.317018838765051,0.333333333333333,0.317018838765051,0.333333333333333,
0.317018838765051,0.333333333333333,0.317018838765051,0.333333333333333,
0.317018838765051,0.333333333333333,0.317018838765051,0.333333333333333,
0.317018838765051,0.333333333333333,0.317018838765051,0.333333333333333,
0.317018838765051,0.333333333333333,0.317018838765051,0.333333333333333,
0.317018838765051,0.333333333333333,0.317018838765051,0.333333333333333,
0.317018838765051,0.333333333333333,0.317018838765051,0.333333333333333),
(1.,0.951056516295154,1.,0.951056516295154,1.,0.951056516295154,1.,0.951056516295154,
1.,0.951056516295154,1.,0.951056516295154,1.,0.951056516295154,1.,0.951056516295154,
1.,0.951056516295154,1.,0.951056516295154,1.,0.951056516295154,1.,0.951056516295154,
1.,0.951056516295154,1.,0.951056516295154,1.,0.951056516295154,1.,0.951056516295154,
1.,0.951056516295154,1.,0.951056516295154,1.,0.951056516295154,1.,0.951056516295154,
1.,0.951056516295154,1.,0.951056516295154,1.,0.951056516295154,1.,0.951056516295154,
1.,0.951056516295154,1.,0.951056516295154,1.,0.951056516295154,1.,0.951056516295154,
1.,0.951056516295154,1.,0.951056516295154,1.,0.951056516295154,1.,0.951056516295154,
1.,0.951056516295154,1.,0.951056516295154,1.,0.951056516295154,1.,0.951056516295154,
1.,0.951056516295154,1.,0.951056516295154,1.,0.951056516295154,1.,0.951056516295154,
1.,0.951056516295154,1.,0.951056516295154,1.,0.951056516295154,1.,0.951056516295154,
1.,0.951056516295154,1.,0.951056516295154,1.,0.951056516295154,1.,0.951056516295154,
1.,0.951056516295154,1.,0.951056516295154,1.,0.951056516295154,1.,0.951056516295154,
1.,0.951056516295154,1.,0.951056516295154,1.,0.951056516295154,1.,0.951056516295154,
1.,0.951056516295154,1.,0.951056516295154,1.,0.951056516295154,1.,0.951056516295154,
1.,0.951056516295154,1.,0.951056516295154,1.,0.951056516295154,1.,0.951056516295154,
1.,0.951056516295154,1.,0.951056516295154,1.,0.951056516295154,1.,0.951056516295154,
1.,0.951056516295154,1.,0.951056516295154,1.,0.951056516295154,1.,0.951056516295154,
1.,0.951056516295154,1.,0.951056516295154,1.,0.951056516295154,1.,0.951056516295154,
1.,0.951056516295154,1.,0.951056516295154,1.,0.951056516295154,1.,0.951056516295154,
1.,0.951056516295154,1.,0.951056516295154,1.,0.951056516295154,1.,0.951056516295154,
1.,0.951056516295154,1.,0.951056516295154,1.,0.951056516295154,1.,0.951056516295154,
1.,0.951056516295154,1.,0.951056516295154,1.,0.951056516295154,1.,0.951056516295154,
1.,0.951056516295154,1.,0.951056516295154,1.,0.951056516295154,1.,0.951056516295154,
1.,0.951056516295154,1.,0.951056516295154,1.,0.951056516295154,1.,0.951056516295154,
1.),(0.333333333333333,0.317018838765051,0.333333333333333,0.317018838765051,
0.333333333333333,0.317018838765051,0.333333333333333,0.317018838765051,
0.333333333333333,0.317018838765051,0.333333333333333,0.317018838765051,
0.333333333333333,0.317018838765051,0.333333333333333,0.317018838765051,
0.333333333333333,0.317018838765051,0.333333333333333,0.317018838765051,
0.333333333333333,0.317018838765051,0.333333333333333,0.317018838765051,
0.333333333333333,0.317018838765051,0.333333333333333,0.317018838765051,
0.333333333333333,0.317018838765051,0.333333333333333,0.317018838765051,
0.333333333333333,0.317018838765051,0.333333333333333,0.317018838765051,
0.333333333333333,0.317018838765051,0.333333333333333,0.317018838765051,
0.333333333333333,0.317018838765051,0.333333333333333,0.317018838765051,
0.333333333333333,0.317018838765051,0.333333333333333,0.317018838765051,
0.333333333333333,0.317018838765051,0.333333333333333,0.317018838765051,
0.333333333333333,0.317018838765051,0.333333333333333,0.317018838765051,
0.333333333333333,0.317018838765051,0.333333333333333,0.317018838765051,
0.333333333333333,0.317018838765051,0.333333333333333,0.317018838765051,
0.333333333333333,0.317018838765051,0.333333333333333,0.317018838765051,
0.333333333333333,0.317018838765051,0.333333333333333,0.317018838765051,
0.333333333333333,0.317018838765051,0.333333333333333,0.317018838765051,
0.333333333333333,0.317018838765051,0.333333333333333,0.317018838765051,
0.333333333333333,0.317018838765051,0.333333333333333,0.317018838765051,
0.333333333333333,0.317018838765051,0.333333333333333,0.317018838765051,
0.333333333333333,0.317018838765051,0.333333333333333,0.317018838765051,
0.333333333333333,0.317018838765051,0.333333333333333,0.317018838765051,
0.333333333333333,0.317018838765051,0.333333333333333,0.317018838765051,
0.333333333333333,0.317018838765051,0.333333333333333,0.317018838765051,
0.333333333333333,0.317018838765051,0.333333333333333,0.317018838765051,
0.333333333333333,0.317018838765051,0.333333333333333,0.317018838765051,
0.333333333333333,0.317018838765051,0.333333333333333,0.317018838765051,
0.333333333333333,0.317018838765051,0.333333333333333,0.317018838765051,
0.333333333333333,0.317018838765051,0.333333333333333,0.317018838765051,
0.333333333333333,0.317018838765051,0.333333333333333,0.317018838765051,
0.333333333333333,0.317018838765051,0.333333333333333,0.317018838765051,
0.333333333333333,0.317018838765051,0.333333333333333,0.317018838765051,
0.333333333333333,0.317018838765051,0.333333333333333,0.317018838765051,
0.333333333333333,0.317018838765051,0.333333333333333,0.317018838765051,
0.333333333333333,0.317018838765051,0.333333333333333,0.317018838765051,
0.333333333333333,0.317018838765051,0.333333333333333,0.317018838765051,
0.333333333333333,0.317018838765051,0.333333333333333,0.317018838765051,
0.333333333333333,0.317018838765051,0.333333333333333,0.317018838765051,
0.333333333333333,0.317018838765051,0.333333333333333,0.317018838765051,
0.333333333333333,0.317018838765051,0.333333333333333,0.317018838765051,
0.333333333333333,0.317018838765051,0.333333333333333,0.317018838765051,
0.333333333333333,0.317018838765051,0.333333333333333,0.317018838765051,
0.333333333333333,0.317018838765051,0.333333333333333,0.317018838765051,
0.333333333333333,0.317018838765051,0.333333333333333,0.317018838765051,
0.333333333333333,0.317018838765051,0.333333333333333,0.317018838765051,
0.333333333333333,0.317018838765051,0.333333333333333,0.317018838765051,
0.333333333333333,0.317018838765051,0.333333333333333,0.317018838765051,
0.333333333333333,0.317018838765051,0.333333333333333,0.317018838765051,
0.333333333333333),(0.333333333333333,0.317018838765051,0.333333333333333,
0.317018838765051,0.333333333333333,0.317018838765051,0.333333333333333,
0.317018838765051,0.333333333333333,0.317018838765051,0.333333333333333,
0.317018838765051,0.333333333333333,0.317018838765051,0.333333333333333,
0.317018838765051,0.333333333333333,0.317018838765051,0.333333333333333,
0.317018838765051,0.333333333333333,0.317018838765051,0.333333333333333,
0.317018838765051,0.333333333333333,0.317018838765051,0.333333333333333,
0.317018838765051,0.333333333333333,0.317018838765051,0.333333333333333,
0.317018838765051,0.333333333333333,0.317018838765051,0.333333333333333,
0.317018838765051,0.333333333333333,0.317018838765051,0.333333333333333,
0.317018838765051,0.333333333333333,0.317018838765051,0.333333333333333,
0.317018838765051,0.333333333333333,0.317018838765051,0.333333333333333,
0.317018838765051,0.333333333333333,0.317018838765051,0.333333333333333,
0.317018838765051,0.333333333333333,0.317018838765051,0.333333333333333,
0.317018838765051,0.333333333333333,0.317018838765051,0.333333333333333,
0.317018838765051,0.333333333333333,0.317018838765051,0.333333333333333,
0.317018838765051,0.333333333333333,0.317018838765051,0.333333333333333,
0.317018838765051,0.333333333333333,0.317018838765051,0.333333333333333,
0.317018838765051,0.333333333333333,0.317018838765051,0.333333333333333,
0.317018838765051,0.333333333333333,0.317018838765051,0.333333333333333,
0.317018838765051,0.333333333333333,0.317018838765051,0.333333333333333,
0.317018838765051,0.333333333333333,0.317018838765051,0.333333333333333,
0.317018838765051,0.333333333333333,0.317018838765051,0.333333333333333,
0.317018838765051,0.333333333333333,0.317018838765051,0.333333333333333,
0.317018838765051,0.333333333333333,0.317018838765051,0.333333333333333,
0.317018838765051,0.333333333333333,0.317018838765051,0.333333333333333,
0.317018838765051,0.333333333333333,0.317018838765051,0.333333333333333,
0.317018838765051,0.333333333333333,0.317018838765051,0.333333333333333,
0.317018838765051,0.333333333333333,0.317018838765051,0.333333333333333,
0.317018838765051,0.333333333333333,0.317018838765051,0.333333333333333,
0.317018838765051,0.333333333333333,0.317018838765051,0.333333333333333,
0.317018838765051,0.333333333333333,0.317018838765051,0.333333333333333,
0.317018838765051,0.333333333333333,0.317018838765051,0.333333333333333,
0.317018838765051,0.333333333333333,0.317018838765051,0.333333333333333,
0.317018838765051,0.333333333333333,0.317018838765051,0.333333333333333,
0.317018838765051,0.333333333333333,0.317018838765051,0.333333333333333,
0.317018838765051,0.333333333333333,0.317018838765051,0.333333333333333,
0.317018838765051,0.333333333333333,0.317018838765051,0.333333333333333,
0.317018838765051,0.333333333333333,0.317018838765051,0.333333333333333,
0.317018838765051,0.333333333333333,0.317018838765051,0.333333333333333,
0.317018838765051,0.333333333333333,0.317018838765051,0.333333333333333,
0.317018838765051,0.333333333333333,0.317018838765051,0.333333333333333,
0.317018838765051,0.333333333333333,0.317018838765051,0.333333333333333,
0.317018838765051,0.333333333333333,0.317018838765051,0.333333333333333,
0.317018838765051,0.333333333333333,0.317018838765051,0.333333333333333,
0.317018838765051,0.333333333333333,0.317018838765051,0.333333333333333,
0.317018838765051,0.333333333333333,0.317018838765051,0.333333333333333,
0.317018838765051,0.333333333333333,0.317018838765051,0.333333333333333,
0.317018838765051,0.333333333333333,0.317018838765051,0.333333333333333,
0.317018838765051,0.333333333333333,0.317018838765051,0.333333333333333,
0.317018838765051,0.333333333333333),(1.,0.951056516295154,1.,0.951056516295154,
1.,0.951056516295154,1.,0.951056516295154,1.,0.951056516295154,1.,0.951056516295154,
1.,0.951056516295154,1.,0.951056516295154,1.,0.951056516295154,1.,0.951056516295154,
1.,0.951056516295154,1.,0.951056516295154,1.,0.951056516295154,1.,0.951056516295154,
1.,0.951056516295154,1.,0.951056516295154,1.,0.951056516295154,1.,0.951056516295154,
1.,0.951056516295154,1.,0.951056516295154,1.,0.951056516295154,1.,0.951056516295154,
1.,0.951056516295154,1.,0.951056516295154,1.,0.951056516295154,1.,0.951056516295154,
1.,0.951056516295154,1.,0.951056516295154,1.,0.951056516295154,1.,0.951056516295154,
1.,0.951056516295154,1.,0.951056516295154,1.,0.951056516295154,1.,0.951056516295154,
1.,0.951056516295154,1.,0.951056516295154,1.,0.951056516295154,1.,0.951056516295154,
1.,0.951056516295154,1.,0.951056516295154,1.,0.951056516295154,1.,0.951056516295154,
1.,0.951056516295154,1.,0.951056516295154,1.,0.951056516295154,1.,0.951056516295154,
1.,0.951056516295154,1.,0.951056516295154,1.,0.951056516295154,1.,0.951056516295154,
1.,0.951056516295154,1.,0.951056516295154,1.,0.951056516295154,1.,0.951056516295154,
1.,0.951056516295154,1.,0.951056516295154,1.,0.951056516295154,1.,0.951056516295154,
1.,0.951056516295154,1.,0.951056516295154,1.,0.951056516295154,1.,0.951056516295154,
1.,0.951056516295154,1.,0.951056516295154,1.,0.951056516295154,1.,0.951056516295154,
1.,0.951056516295154,1.,0.951056516295154,1.,0.951056516295154,1.,0.951056516295154,
1.,0.951056516295154,1.,0.951056516295154,1.,0.951056516295154,1.,0.951056516295154,
1.,0.951056516295154,1.,0.951056516295154,1.,0.951056516295154,1.,0.951056516295154,
1.,0.951056516295154,1.,0.951056516295154,1.,0.951056516295154,1.,0.951056516295154,
1.,0.951056516295154,1.,0.951056516295154,1.,0.951056516295154,1.,0.951056516295154,
1.,0.951056516295154,1.,0.951056516295154,1.,0.951056516295154,1.,0.951056516295154,
1.,0.951056516295154,1.,0.951056516295154,1.,0.951056516295154,1.,0.951056516295154,
1.,0.951056516295154,1.,0.951056516295154,1.,0.951056516295154,1.,0.951056516295154,
1.,0.951056516295154,1.,0.951056516295154,1.)))
REPRESENTATION_ITEM('')
SURFACE()
);
#100=SHAPE_REPRESENTATION_RELATIONSHIP('SRR','None',#7668,#109);
#109=ADVANCED_BREP_SHAPE_REPRESENTATION('',(#139),#7621);
#118=STYLED_ITEM('',(#7722),#139);
#139=MANIFOLD_SOLID_BREP('Body1',#2416);
#208=PLANE('',#2603);
#209=PLANE('',#2605);
#210=PLANE('',#2607);
#342=FACE_OUTER_BOUND('',#507,.T.);
#343=FACE_OUTER_BOUND('',#508,.T.);
#344=FACE_OUTER_BOUND('',#509,.T.);
#345=FACE_OUTER_BOUND('',#510,.T.);
#346=FACE_OUTER_BOUND('',#511,.T.);
#507=EDGE_LOOP('',(#1747,#1748,#1749,#1750,#1751));
#508=EDGE_LOOP('',(#1752,#1753,#1754));
#509=EDGE_LOOP('',(#1755,#1756));
#510=EDGE_LOOP('',(#1757,#1758,#1759,#1760,#1761));
#511=EDGE_LOOP('',(#1762,#1763,#1764));
#675=CIRCLE('',#2601,0.500000000000003);
#676=CIRCLE('',#2602,0.499999999999999);
#677=CIRCLE('',#2604,0.499999999999999);
#678=CIRCLE('',#2606,0.500000000000003);
#838=LINE('',#5658,#994);
#994=VECTOR('',#3039,1000.);
#1157=VERTEX_POINT('',#5231);
#1158=VERTEX_POINT('',#5232);
#1159=VERTEX_POINT('',#5251);
#1160=VERTEX_POINT('',#5451);
#1161=VERTEX_POINT('',#5453);
#1162=VERTEX_POINT('',#5657);
#1368=EDGE_CURVE('',#1157,#1158,#93,.T.);
#1369=EDGE_CURVE('',#1157,#1159,#91,.T.);
#1370=EDGE_CURVE('',#1159,#1160,#675,.T.);
#1371=EDGE_CURVE('',#1161,#1160,#92,.T.);
#1372=EDGE_CURVE('',#1161,#1158,#676,.T.);
#1373=EDGE_CURVE('',#1158,#1162,#838,.T.);
#1374=EDGE_CURVE('',#1162,#1161,#677,.T.);
#1375=EDGE_CURVE('',#1160,#1159,#678,.T.);
#1376=EDGE_CURVE('',#1162,#1157,#94,.T.);
#1747=ORIENTED_EDGE('',*,*,#1368,.F.);
#1748=ORIENTED_EDGE('',*,*,#1369,.T.);
#1749=ORIENTED_EDGE('',*,*,#1370,.T.);
#1750=ORIENTED_EDGE('',*,*,#1371,.F.);
#1751=ORIENTED_EDGE('',*,*,#1372,.T.);
#1752=ORIENTED_EDGE('',*,*,#1373,.F.);
#1753=ORIENTED_EDGE('',*,*,#1372,.F.);
#1754=ORIENTED_EDGE('',*,*,#1374,.F.);
#1755=ORIENTED_EDGE('',*,*,#1375,.F.);
#1756=ORIENTED_EDGE('',*,*,#1370,.F.);
#1757=ORIENTED_EDGE('',*,*,#1369,.F.);
#1758=ORIENTED_EDGE('',*,*,#1376,.F.);
#1759=ORIENTED_EDGE('',*,*,#1374,.T.);
#1760=ORIENTED_EDGE('',*,*,#1371,.T.);
#1761=ORIENTED_EDGE('',*,*,#1375,.T.);
#1762=ORIENTED_EDGE('',*,*,#1373,.T.);
#1763=ORIENTED_EDGE('',*,*,#1376,.T.);
#1764=ORIENTED_EDGE('',*,*,#1368,.T.);
#2293=ADVANCED_FACE('',(#342),#95,.T.);
#2294=ADVANCED_FACE('',(#343),#208,.T.);
#2295=ADVANCED_FACE('',(#344),#209,.F.);
#2296=ADVANCED_FACE('',(#345),#96,.T.);
#2297=ADVANCED_FACE('',(#346),#210,.F.);
#2416=CLOSED_SHELL('',(#2293,#2294,#2295,#2296,#2297));
#2600=AXIS2_PLACEMENT_3D('',#3823,#3031,#3032);
#2601=AXIS2_PLACEMENT_3D('',#5452,#3033,#3034);
#2602=AXIS2_PLACEMENT_3D('',#5655,#3035,#3036);
#2603=AXIS2_PLACEMENT_3D('',#5656,#3037,#3038);
#2604=AXIS2_PLACEMENT_3D('',#5659,#3040,#3041);
#2605=AXIS2_PLACEMENT_3D('',#5660,#3042,#3043);
#2606=AXIS2_PLACEMENT_3D('',#5661,#3044,#3045);
#2607=AXIS2_PLACEMENT_3D('',#7087,#3046,#3047);
#3031=DIRECTION('axis',(0.,0.,1.));
#3032=DIRECTION('refdir',(1.,0.,0.));
#3033=DIRECTION('center_axis',(1.02811330220411E-14,-0.112954554410665,
0.993600155312935));
#3034=DIRECTION('ref_axis',(2.38360928778941E-29,0.993600155312935,0.112954554410665));
#3035=DIRECTION('center_axis',(-1.02811330220411E-14,0.112954554410665,
-0.993600155312935));
#3036=DIRECTION('ref_axis',(1.8514835708046E-30,0.993600155312935,0.112954554410665));
#3037=DIRECTION('center_axis',(1.04703450427522E-14,-0.112954554410665,
0.993600155312935));
#3038=DIRECTION('ref_axis',(-2.63248751403759E-32,-0.993600155312935,-0.112954554410665));
#3039=DIRECTION('',(-1.,0.,1.053778523158E-14));
#3040=DIRECTION('center_axis',(-1.02811330220411E-14,0.112954554410665,
-0.993600155312935));
#3041=DIRECTION('ref_axis',(1.8514835708046E-30,0.993600155312935,0.112954554410665));
#3042=DIRECTION('center_axis',(1.02744001254975E-14,-0.112954554410666,
0.993600155312935));
#3043=DIRECTION('ref_axis',(-6.45044998851022E-32,-0.993600155312935,-0.112954554410666));
#3044=DIRECTION('center_axis',(1.02811330220411E-14,-0.112954554410665,
0.993600155312935));
#3045=DIRECTION('ref_axis',(2.38360928778941E-29,0.993600155312935,0.112954554410665));
#3046=DIRECTION('center_axis',(0.,1.,0.));
#3047=DIRECTION('ref_axis',(0.,0.,1.));
#3823=CARTESIAN_POINT('',(0.,0.,0.));
#3824=CARTESIAN_POINT('Ctrl Pts',(-3.5,15.4968000776565,0.0564772772053689));
#3825=CARTESIAN_POINT('Ctrl Pts',(-3.51835057975363,15.6218000776565,-1.0807416596098));
#3826=CARTESIAN_POINT('Ctrl Pts',(-2.86475599094327,15.7468000776565,-2.01155730596849));
#3827=CARTESIAN_POINT('Ctrl Pts',(-2.2111614021329,15.8718000776565,-2.94237295232717));
#3828=CARTESIAN_POINT('Ctrl Pts',(-1.13527256282109,15.9968000776565,-3.31124536858055));
#3829=CARTESIAN_POINT('Ctrl Pts',(-0.0593837235092786,16.1218000776565,
-3.68011778483394));
#3830=CARTESIAN_POINT('Ctrl Pts',(1.02784639780354,16.2468000776565,-3.34615024548552));
#3831=CARTESIAN_POINT('Ctrl Pts',(2.11507651911636,16.3718000776565,-3.01218270613711));
#3832=CARTESIAN_POINT('Ctrl Pts',(2.79836296968137,16.4968000776565,-2.10293946007882));
#3833=CARTESIAN_POINT('Ctrl Pts',(3.48164942024637,16.6218000776565,-1.19369621402054));
#3834=CARTESIAN_POINT('Ctrl Pts',(3.5,16.7468000776565,-0.0564772772053694));
#3835=CARTESIAN_POINT('Ctrl Pts',(3.51835057975363,16.8718000776565,1.0807416596098));
#3836=CARTESIAN_POINT('Ctrl Pts',(2.86475599094327,16.9968000776565,2.01155730596849));
#3837=CARTESIAN_POINT('Ctrl Pts',(2.2111614021329,17.1218000776565,2.94237295232717));
#3838=CARTESIAN_POINT('Ctrl Pts',(1.13527256282109,17.2468000776565,3.31124536858055));
#3839=CARTESIAN_POINT('Ctrl Pts',(0.0593837235092791,17.3718000776565,3.68011778483394));
#3840=CARTESIAN_POINT('Ctrl Pts',(-1.02784639780354,17.4968000776565,3.34615024548552));
#3841=CARTESIAN_POINT('Ctrl Pts',(-2.11507651911636,17.6218000776565,3.01218270613711));
#3842=CARTESIAN_POINT('Ctrl Pts',(-2.79836296968137,17.7468000776565,2.10293946007882));
#3843=CARTESIAN_POINT('Ctrl Pts',(-3.48164942024637,17.8718000776565,1.19369621402054));
#3844=CARTESIAN_POINT('Ctrl Pts',(-3.5,17.9968000776565,0.0564772772053689));
#3845=CARTESIAN_POINT('Ctrl Pts',(-3.51835057975363,18.1218000776565,-1.0807416596098));
#3846=CARTESIAN_POINT('Ctrl Pts',(-2.86475599094327,18.2468000776565,-2.01155730596849));
#3847=CARTESIAN_POINT('Ctrl Pts',(-2.2111614021329,18.3718000776565,-2.94237295232717));
#3848=CARTESIAN_POINT('Ctrl Pts',(-1.13527256282109,18.4968000776565,-3.31124536858055));
#3849=CARTESIAN_POINT('Ctrl Pts',(-0.0593837235092786,18.6218000776565,
-3.68011778483394));
#3850=CARTESIAN_POINT('Ctrl Pts',(1.02784639780354,18.7468000776565,-3.34615024548552));
#3851=CARTESIAN_POINT('Ctrl Pts',(2.11507651911636,18.8718000776565,-3.01218270613711));
#3852=CARTESIAN_POINT('Ctrl Pts',(2.79836296968137,18.9968000776565,-2.10293946007882));
#3853=CARTESIAN_POINT('Ctrl Pts',(3.48164942024637,19.1218000776565,-1.19369621402054));
#3854=CARTESIAN_POINT('Ctrl Pts',(3.5,19.2468000776565,-0.0564772772053694));
#3855=CARTESIAN_POINT('Ctrl Pts',(3.51835057975363,19.3718000776565,1.0807416596098));
#3856=CARTESIAN_POINT('Ctrl Pts',(2.86475599094327,19.4968000776565,2.01155730596849));
#3857=CARTESIAN_POINT('Ctrl Pts',(2.2111614021329,19.6218000776565,2.94237295232717));
#3858=CARTESIAN_POINT('Ctrl Pts',(1.13527256282109,19.7468000776565,3.31124536858055));
#3859=CARTESIAN_POINT('Ctrl Pts',(0.0593837235092791,19.8718000776565,3.68011778483394));
#3860=CARTESIAN_POINT('Ctrl Pts',(-1.02784639780354,19.9968000776565,3.34615024548552));
#3861=CARTESIAN_POINT('Ctrl Pts',(-2.11507651911636,20.1218000776565,3.01218270613711));
#3862=CARTESIAN_POINT('Ctrl Pts',(-2.79836296968137,20.2468000776565,2.10293946007882));
#3863=CARTESIAN_POINT('Ctrl Pts',(-3.48164942024637,20.3718000776565,1.19369621402054));
#3864=CARTESIAN_POINT('Ctrl Pts',(-3.5,20.4968000776565,0.0564772772053689));
#3865=CARTESIAN_POINT('Ctrl Pts',(-3.51835057975363,20.6218000776565,-1.0807416596098));
#3866=CARTESIAN_POINT('Ctrl Pts',(-2.86475599094327,20.7468000776565,-2.01155730596849));
#3867=CARTESIAN_POINT('Ctrl Pts',(-2.2111614021329,20.8718000776565,-2.94237295232717));
#3868=CARTESIAN_POINT('Ctrl Pts',(-1.13527256282109,20.9968000776565,-3.31124536858055));
#3869=CARTESIAN_POINT('Ctrl Pts',(-0.0593837235092786,21.1218000776565,
-3.68011778483394));
#3870=CARTESIAN_POINT('Ctrl Pts',(1.02784639780354,21.2468000776565,-3.34615024548552));
#3871=CARTESIAN_POINT('Ctrl Pts',(2.11507651911636,21.3718000776565,-3.01218270613711));
#3872=CARTESIAN_POINT('Ctrl Pts',(2.79836296968137,21.4968000776565,-2.10293946007882));
#3873=CARTESIAN_POINT('Ctrl Pts',(3.48164942024637,21.6218000776565,-1.19369621402054));
#3874=CARTESIAN_POINT('Ctrl Pts',(3.5,21.7468000776565,-0.0564772772053694));
#3875=CARTESIAN_POINT('Ctrl Pts',(3.51835057975363,21.8718000776565,1.0807416596098));
#3876=CARTESIAN_POINT('Ctrl Pts',(2.86475599094327,21.9968000776565,2.01155730596849));
#3877=CARTESIAN_POINT('Ctrl Pts',(2.2111614021329,22.1218000776565,2.94237295232717));
#3878=CARTESIAN_POINT('Ctrl Pts',(1.13527256282109,22.2468000776565,3.31124536858055));
#3879=CARTESIAN_POINT('Ctrl Pts',(0.0593837235092791,22.3718000776565,3.68011778483394));
#3880=CARTESIAN_POINT('Ctrl Pts',(-1.02784639780354,22.4968000776565,3.34615024548552));
#3881=CARTESIAN_POINT('Ctrl Pts',(-2.11507651911636,22.6218000776565,3.01218270613711));
#3882=CARTESIAN_POINT('Ctrl Pts',(-2.79836296968137,22.7468000776565,2.10293946007882));
#3883=CARTESIAN_POINT('Ctrl Pts',(-3.48164942024637,22.8718000776565,1.19369621402054));
#3884=CARTESIAN_POINT('Ctrl Pts',(-3.5,22.9968000776565,0.0564772772053689));
#3885=CARTESIAN_POINT('Ctrl Pts',(-3.51835057975363,23.1218000776565,-1.0807416596098));
#3886=CARTESIAN_POINT('Ctrl Pts',(-2.86475599094327,23.2468000776565,-2.01155730596849));
#3887=CARTESIAN_POINT('Ctrl Pts',(-2.2111614021329,23.3718000776565,-2.94237295232717));
#3888=CARTESIAN_POINT('Ctrl Pts',(-1.13527256282109,23.4968000776565,-3.31124536858055));
#3889=CARTESIAN_POINT('Ctrl Pts',(-0.0593837235092786,23.6218000776565,
-3.68011778483394));
#3890=CARTESIAN_POINT('Ctrl Pts',(1.02784639780354,23.7468000776565,-3.34615024548552));
#3891=CARTESIAN_POINT('Ctrl Pts',(2.11507651911636,23.8718000776565,-3.01218270613711));
#3892=CARTESIAN_POINT('Ctrl Pts',(2.79836296968137,23.9968000776565,-2.10293946007882));
#3893=CARTESIAN_POINT('Ctrl Pts',(3.48164942024637,24.1218000776565,-1.19369621402054));
#3894=CARTESIAN_POINT('Ctrl Pts',(3.5,24.2468000776565,-0.0564772772053694));
#3895=CARTESIAN_POINT('Ctrl Pts',(3.51835057975363,24.3718000776565,1.0807416596098));
#3896=CARTESIAN_POINT('Ctrl Pts',(2.86475599094327,24.4968000776565,2.01155730596849));
#3897=CARTESIAN_POINT('Ctrl Pts',(2.2111614021329,24.6218000776565,2.94237295232717));
#3898=CARTESIAN_POINT('Ctrl Pts',(1.13527256282109,24.7468000776565,3.31124536858055));
#3899=CARTESIAN_POINT('Ctrl Pts',(0.0593837235092791,24.8718000776565,3.68011778483394));
#3900=CARTESIAN_POINT('Ctrl Pts',(-1.02784639780354,24.9968000776565,3.34615024548552));
#3901=CARTESIAN_POINT('Ctrl Pts',(-2.11507651911636,25.1218000776565,3.01218270613711));
#3902=CARTESIAN_POINT('Ctrl Pts',(-2.79836296968137,25.2468000776565,2.10293946007882));
#3903=CARTESIAN_POINT('Ctrl Pts',(-3.48164942024637,25.3718000776565,1.19369621402054));
#3904=CARTESIAN_POINT('Ctrl Pts',(-3.5,25.4968000776565,0.0564772772053689));
#3905=CARTESIAN_POINT('Ctrl Pts',(-3.51835057975363,25.6218000776565,-1.0807416596098));
#3906=CARTESIAN_POINT('Ctrl Pts',(-2.86475599094327,25.7468000776565,-2.01155730596849));
#3907=CARTESIAN_POINT('Ctrl Pts',(-2.2111614021329,25.8718000776565,-2.94237295232717));
#3908=CARTESIAN_POINT('Ctrl Pts',(-1.13527256282109,25.9968000776565,-3.31124536858055));
#3909=CARTESIAN_POINT('Ctrl Pts',(-0.0593837235092786,26.1218000776565,
-3.68011778483394));
#3910=CARTESIAN_POINT('Ctrl Pts',(1.02784639780354,26.2468000776565,-3.34615024548552));
#3911=CARTESIAN_POINT('Ctrl Pts',(2.11507651911636,26.3718000776565,-3.01218270613711));
#3912=CARTESIAN_POINT('Ctrl Pts',(2.79836296968137,26.4968000776565,-2.10293946007882));
#3913=CARTESIAN_POINT('Ctrl Pts',(3.48164942024637,26.6218000776565,-1.19369621402054));
#3914=CARTESIAN_POINT('Ctrl Pts',(3.5,26.7468000776565,-0.0564772772053694));
#3915=CARTESIAN_POINT('Ctrl Pts',(3.51835057975363,26.8718000776565,1.0807416596098));
#3916=CARTESIAN_POINT('Ctrl Pts',(2.86475599094327,26.9968000776565,2.01155730596849));
#3917=CARTESIAN_POINT('Ctrl Pts',(2.2111614021329,27.1218000776565,2.94237295232717));
#3918=CARTESIAN_POINT('Ctrl Pts',(1.13527256282109,27.2468000776565,3.31124536858055));
#3919=CARTESIAN_POINT('Ctrl Pts',(0.0593837235092791,27.3718000776565,3.68011778483394));
#3920=CARTESIAN_POINT('Ctrl Pts',(-1.02784639780354,27.4968000776565,3.34615024548552));
#3921=CARTESIAN_POINT('Ctrl Pts',(-2.11507651911636,27.6218000776565,3.01218270613711));
#3922=CARTESIAN_POINT('Ctrl Pts',(-2.79836296968137,27.7468000776565,2.10293946007882));
#3923=CARTESIAN_POINT('Ctrl Pts',(-3.48164942024637,27.8718000776565,1.19369621402054));
#3924=CARTESIAN_POINT('Ctrl Pts',(-3.5,27.9968000776565,0.0564772772053689));
#3925=CARTESIAN_POINT('Ctrl Pts',(-3.51835057975363,28.1218000776565,-1.0807416596098));
#3926=CARTESIAN_POINT('Ctrl Pts',(-2.86475599094327,28.2468000776565,-2.01155730596849));
#3927=CARTESIAN_POINT('Ctrl Pts',(-2.2111614021329,28.3718000776565,-2.94237295232717));
#3928=CARTESIAN_POINT('Ctrl Pts',(-1.13527256282109,28.4968000776565,-3.31124536858055));
#3929=CARTESIAN_POINT('Ctrl Pts',(-0.0593837235092786,28.6218000776565,
-3.68011778483394));
#3930=CARTESIAN_POINT('Ctrl Pts',(1.02784639780354,28.7468000776565,-3.34615024548552));
#3931=CARTESIAN_POINT('Ctrl Pts',(2.11507651911636,28.8718000776565,-3.01218270613711));
#3932=CARTESIAN_POINT('Ctrl Pts',(2.79836296968137,28.9968000776565,-2.10293946007882));
#3933=CARTESIAN_POINT('Ctrl Pts',(3.48164942024637,29.1218000776565,-1.19369621402054));
#3934=CARTESIAN_POINT('Ctrl Pts',(3.5,29.2468000776565,-0.0564772772053694));
#3935=CARTESIAN_POINT('Ctrl Pts',(3.51835057975363,29.3718000776565,1.0807416596098));
#3936=CARTESIAN_POINT('Ctrl Pts',(2.86475599094327,29.4968000776565,2.01155730596849));
#3937=CARTESIAN_POINT('Ctrl Pts',(2.2111614021329,29.6218000776565,2.94237295232717));
#3938=CARTESIAN_POINT('Ctrl Pts',(1.13527256282109,29.7468000776565,3.31124536858055));
#3939=CARTESIAN_POINT('Ctrl Pts',(0.0593837235092791,29.8718000776565,3.68011778483394));
#3940=CARTESIAN_POINT('Ctrl Pts',(-1.02784639780354,29.9968000776565,3.34615024548552));
#3941=CARTESIAN_POINT('Ctrl Pts',(-2.11507651911636,30.1218000776565,3.01218270613711));
#3942=CARTESIAN_POINT('Ctrl Pts',(-2.79836296968137,30.2468000776565,2.10293946007882));
#3943=CARTESIAN_POINT('Ctrl Pts',(-3.48164942024637,30.3718000776565,1.19369621402054));
#3944=CARTESIAN_POINT('Ctrl Pts',(-3.5,30.4968000776565,0.0564772772053689));
#3945=CARTESIAN_POINT('Ctrl Pts',(-3.51835057975363,30.6218000776565,-1.0807416596098));
#3946=CARTESIAN_POINT('Ctrl Pts',(-2.86475599094327,30.7468000776565,-2.01155730596849));
#3947=CARTESIAN_POINT('Ctrl Pts',(-2.2111614021329,30.8718000776565,-2.94237295232717));
#3948=CARTESIAN_POINT('Ctrl Pts',(-1.13527256282109,30.9968000776565,-3.31124536858055));
#3949=CARTESIAN_POINT('Ctrl Pts',(-0.0593837235092786,31.1218000776565,
-3.68011778483394));
#3950=CARTESIAN_POINT('Ctrl Pts',(1.02784639780354,31.2468000776565,-3.34615024548552));
#3951=CARTESIAN_POINT('Ctrl Pts',(2.11507651911636,31.3718000776565,-3.01218270613711));
#3952=CARTESIAN_POINT('Ctrl Pts',(2.79836296968137,31.4968000776565,-2.10293946007882));
#3953=CARTESIAN_POINT('Ctrl Pts',(3.48164942024637,31.6218000776565,-1.19369621402054));
#3954=CARTESIAN_POINT('Ctrl Pts',(3.5,31.7468000776565,-0.0564772772053694));
#3955=CARTESIAN_POINT('Ctrl Pts',(3.51835057975363,31.8718000776565,1.0807416596098));
#3956=CARTESIAN_POINT('Ctrl Pts',(2.86475599094327,31.9968000776565,2.01155730596849));
#3957=CARTESIAN_POINT('Ctrl Pts',(2.2111614021329,32.1218000776565,2.94237295232717));
#3958=CARTESIAN_POINT('Ctrl Pts',(1.13527256282109,32.2468000776565,3.31124536858055));
#3959=CARTESIAN_POINT('Ctrl Pts',(0.0593837235092791,32.3718000776565,3.68011778483394));
#3960=CARTESIAN_POINT('Ctrl Pts',(-1.02784639780354,32.4968000776565,3.34615024548552));
#3961=CARTESIAN_POINT('Ctrl Pts',(-2.11507651911636,32.6218000776565,3.01218270613711));
#3962=CARTESIAN_POINT('Ctrl Pts',(-2.79836296968137,32.7468000776565,2.10293946007882));
#3963=CARTESIAN_POINT('Ctrl Pts',(-3.48164942024637,32.8718000776565,1.19369621402054));
#3964=CARTESIAN_POINT('Ctrl Pts',(-3.5,32.9968000776565,0.0564772772053689));
#3965=CARTESIAN_POINT('Ctrl Pts',(-3.51835057975363,33.1218000776565,-1.0807416596098));
#3966=CARTESIAN_POINT('Ctrl Pts',(-2.86475599094327,33.2468000776565,-2.01155730596849));
#3967=CARTESIAN_POINT('Ctrl Pts',(-2.2111614021329,33.3718000776565,-2.94237295232717));
#3968=CARTESIAN_POINT('Ctrl Pts',(-1.13527256282109,33.4968000776565,-3.31124536858055));
#3969=CARTESIAN_POINT('Ctrl Pts',(-0.0593837235092786,33.6218000776565,
-3.68011778483394));
#3970=CARTESIAN_POINT('Ctrl Pts',(1.02784639780354,33.7468000776565,-3.34615024548552));
#3971=CARTESIAN_POINT('Ctrl Pts',(2.11507651911636,33.8718000776565,-3.01218270613711));
#3972=CARTESIAN_POINT('Ctrl Pts',(2.79836296968137,33.9968000776565,-2.10293946007882));
#3973=CARTESIAN_POINT('Ctrl Pts',(3.48164942024637,34.1218000776565,-1.19369621402054));
#3974=CARTESIAN_POINT('Ctrl Pts',(3.5,34.2468000776565,-0.0564772772053694));
#3975=CARTESIAN_POINT('Ctrl Pts',(3.51835057975363,34.3718000776565,1.0807416596098));
#3976=CARTESIAN_POINT('Ctrl Pts',(2.86475599094327,34.4968000776565,2.01155730596849));
#3977=CARTESIAN_POINT('Ctrl Pts',(2.2111614021329,34.6218000776565,2.94237295232717));
#3978=CARTESIAN_POINT('Ctrl Pts',(1.13527256282109,34.7468000776565,3.31124536858055));
#3979=CARTESIAN_POINT('Ctrl Pts',(0.0593837235092791,34.8718000776565,3.68011778483394));
#3980=CARTESIAN_POINT('Ctrl Pts',(-1.02784639780354,34.9968000776565,3.34615024548552));
#3981=CARTESIAN_POINT('Ctrl Pts',(-2.11507651911636,35.1218000776565,3.01218270613711));
#3982=CARTESIAN_POINT('Ctrl Pts',(-2.79836296968137,35.2468000776565,2.10293946007882));
#3983=CARTESIAN_POINT('Ctrl Pts',(-3.48164942024637,35.3718000776565,1.19369621402054));
#3984=CARTESIAN_POINT('Ctrl Pts',(-3.5,35.4968000776565,0.0564772772053689));
#3985=CARTESIAN_POINT('Ctrl Pts',(-3.51835057975363,35.6218000776565,-1.0807416596098));
#3986=CARTESIAN_POINT('Ctrl Pts',(-2.86475599094327,35.7468000776565,-2.01155730596849));
#3987=CARTESIAN_POINT('Ctrl Pts',(-2.2111614021329,35.8718000776565,-2.94237295232717));
#3988=CARTESIAN_POINT('Ctrl Pts',(-1.13527256282109,35.9968000776565,-3.31124536858055));
#3989=CARTESIAN_POINT('Ctrl Pts',(-0.0593837235092786,36.1218000776565,
-3.68011778483394));
#3990=CARTESIAN_POINT('Ctrl Pts',(1.02784639780354,36.2468000776565,-3.34615024548552));
#3991=CARTESIAN_POINT('Ctrl Pts',(2.11507651911636,36.3718000776565,-3.01218270613711));
#3992=CARTESIAN_POINT('Ctrl Pts',(2.79836296968137,36.4968000776565,-2.10293946007882));
#3993=CARTESIAN_POINT('Ctrl Pts',(3.48164942024637,36.6218000776565,-1.19369621402054));
#3994=CARTESIAN_POINT('Ctrl Pts',(3.5,36.7468000776565,-0.0564772772053694));
#3995=CARTESIAN_POINT('Ctrl Pts',(3.51835057975363,36.8718000776565,1.0807416596098));
#3996=CARTESIAN_POINT('Ctrl Pts',(2.86475599094327,36.9968000776565,2.01155730596849));
#3997=CARTESIAN_POINT('Ctrl Pts',(2.2111614021329,37.1218000776565,2.94237295232717));
#3998=CARTESIAN_POINT('Ctrl Pts',(1.13527256282109,37.2468000776565,3.31124536858055));
#3999=CARTESIAN_POINT('Ctrl Pts',(0.0593837235092791,37.3718000776565,3.68011778483394));
#4000=CARTESIAN_POINT('Ctrl Pts',(-1.02784639780354,37.4968000776565,3.34615024548552));
#4001=CARTESIAN_POINT('Ctrl Pts',(-2.11507651911636,37.6218000776565,3.01218270613711));
#4002=CARTESIAN_POINT('Ctrl Pts',(-2.79836296968137,37.7468000776565,2.10293946007882));
#4003=CARTESIAN_POINT('Ctrl Pts',(-3.48164942024637,37.8718000776565,1.19369621402054));
#4004=CARTESIAN_POINT('Ctrl Pts',(-3.5,37.9968000776565,0.0564772772053689));
#4005=CARTESIAN_POINT('Ctrl Pts',(-3.51835057975363,38.1218000776565,-1.0807416596098));
#4006=CARTESIAN_POINT('Ctrl Pts',(-2.86475599094327,38.2468000776565,-2.01155730596849));
#4007=CARTESIAN_POINT('Ctrl Pts',(-2.2111614021329,38.3718000776565,-2.94237295232717));
#4008=CARTESIAN_POINT('Ctrl Pts',(-1.13527256282109,38.4968000776565,-3.31124536858055));
#4009=CARTESIAN_POINT('Ctrl Pts',(-0.0593837235092786,38.6218000776565,
-3.68011778483394));
#4010=CARTESIAN_POINT('Ctrl Pts',(1.02784639780354,38.7468000776565,-3.34615024548552));
#4011=CARTESIAN_POINT('Ctrl Pts',(2.11507651911636,38.8718000776565,-3.01218270613711));
#4012=CARTESIAN_POINT('Ctrl Pts',(2.79836296968137,38.9968000776565,-2.10293946007882));
#4013=CARTESIAN_POINT('Ctrl Pts',(3.48164942024637,39.1218000776565,-1.19369621402054));
#4014=CARTESIAN_POINT('Ctrl Pts',(3.5,39.2468000776565,-0.0564772772053694));
#4015=CARTESIAN_POINT('Ctrl Pts',(3.51835057975363,39.3718000776565,1.0807416596098));
#4016=CARTESIAN_POINT('Ctrl Pts',(2.86475599094327,39.4968000776565,2.01155730596849));
#4017=CARTESIAN_POINT('Ctrl Pts',(2.2111614021329,39.6218000776565,2.94237295232717));
#4018=CARTESIAN_POINT('Ctrl Pts',(1.13527256282109,39.7468000776565,3.31124536858055));
#4019=CARTESIAN_POINT('Ctrl Pts',(0.0593837235092791,39.8718000776565,3.68011778483394));
#4020=CARTESIAN_POINT('Ctrl Pts',(-1.02784639780354,39.9968000776565,3.34615024548552));
#4021=CARTESIAN_POINT('Ctrl Pts',(-2.11507651911636,40.1218000776565,3.01218270613711));
#4022=CARTESIAN_POINT('Ctrl Pts',(-2.79836296968137,40.2468000776565,2.10293946007882));
#4023=CARTESIAN_POINT('Ctrl Pts',(-3.48164942024637,40.3718000776565,1.19369621402054));
#4024=CARTESIAN_POINT('Ctrl Pts',(-3.5,40.4968000776565,0.0564772772053689));
#4025=CARTESIAN_POINT('Ctrl Pts',(-2.5,15.4968000776565,0.0564772772053586));
#4026=CARTESIAN_POINT('Ctrl Pts',(-2.51835057975363,15.6218000776565,-0.755821963376908));
#4027=CARTESIAN_POINT('Ctrl Pts',(-2.05573899656831,15.7468000776565,-1.42377205367602));
#4028=CARTESIAN_POINT('Ctrl Pts',(-1.593127413383,15.8718000776565,-2.09172214397514));
#4029=CARTESIAN_POINT('Ctrl Pts',(-0.826255568446133,15.9968000776565,-2.3601888522854));
#4030=CARTESIAN_POINT('Ctrl Pts',(-0.0593837235092677,16.1218000776565,
-2.62865556059567));
#4031=CARTESIAN_POINT('Ctrl Pts',(0.718829403428605,16.2468000776565,-2.39509372919037));
#4032=CARTESIAN_POINT('Ctrl Pts',(1.49704253036648,16.3718000776565,-2.16153189778506));
#4033=CARTESIAN_POINT('Ctrl Pts',(1.98934597530643,16.4968000776565,-1.51515420778634));
#4034=CARTESIAN_POINT('Ctrl Pts',(2.48164942024637,16.6218000776565,-0.868776517787625));
#4035=CARTESIAN_POINT('Ctrl Pts',(2.5,16.7468000776565,-0.0564772772053589));
#4036=CARTESIAN_POINT('Ctrl Pts',(2.51835057975363,16.8718000776565,0.755821963376907));
#4037=CARTESIAN_POINT('Ctrl Pts',(2.05573899656831,16.9968000776565,1.42377205367602));
#4038=CARTESIAN_POINT('Ctrl Pts',(1.593127413383,17.1218000776565,2.09172214397514));
#4039=CARTESIAN_POINT('Ctrl Pts',(0.826255568446133,17.2468000776565,2.3601888522854));
#4040=CARTESIAN_POINT('Ctrl Pts',(0.059383723509268,17.3718000776565,2.62865556059567));
#4041=CARTESIAN_POINT('Ctrl Pts',(-0.718829403428604,17.4968000776565,2.39509372919037));
#4042=CARTESIAN_POINT('Ctrl Pts',(-1.49704253036648,17.6218000776565,2.16153189778506));
#4043=CARTESIAN_POINT('Ctrl Pts',(-1.98934597530643,17.7468000776565,1.51515420778634));
#4044=CARTESIAN_POINT('Ctrl Pts',(-2.48164942024637,17.8718000776565,0.868776517787626));
#4045=CARTESIAN_POINT('Ctrl Pts',(-2.5,17.9968000776565,0.0564772772053586));
#4046=CARTESIAN_POINT('Ctrl Pts',(-2.51835057975363,18.1218000776565,-0.755821963376908));
#4047=CARTESIAN_POINT('Ctrl Pts',(-2.05573899656831,18.2468000776565,-1.42377205367602));
#4048=CARTESIAN_POINT('Ctrl Pts',(-1.593127413383,18.3718000776565,-2.09172214397514));
#4049=CARTESIAN_POINT('Ctrl Pts',(-0.826255568446133,18.4968000776565,-2.3601888522854));
#4050=CARTESIAN_POINT('Ctrl Pts',(-0.0593837235092677,18.6218000776565,
-2.62865556059567));
#4051=CARTESIAN_POINT('Ctrl Pts',(0.718829403428605,18.7468000776565,-2.39509372919037));
#4052=CARTESIAN_POINT('Ctrl Pts',(1.49704253036648,18.8718000776565,-2.16153189778506));
#4053=CARTESIAN_POINT('Ctrl Pts',(1.98934597530643,18.9968000776565,-1.51515420778634));
#4054=CARTESIAN_POINT('Ctrl Pts',(2.48164942024637,19.1218000776565,-0.868776517787625));
#4055=CARTESIAN_POINT('Ctrl Pts',(2.5,19.2468000776565,-0.0564772772053589));
#4056=CARTESIAN_POINT('Ctrl Pts',(2.51835057975363,19.3718000776565,0.755821963376907));
#4057=CARTESIAN_POINT('Ctrl Pts',(2.05573899656831,19.4968000776565,1.42377205367602));
#4058=CARTESIAN_POINT('Ctrl Pts',(1.593127413383,19.6218000776565,2.09172214397514));
#4059=CARTESIAN_POINT('Ctrl Pts',(0.826255568446133,19.7468000776565,2.3601888522854));
#4060=CARTESIAN_POINT('Ctrl Pts',(0.059383723509268,19.8718000776565,2.62865556059567));
#4061=CARTESIAN_POINT('Ctrl Pts',(-0.718829403428604,19.9968000776565,2.39509372919037));
#4062=CARTESIAN_POINT('Ctrl Pts',(-1.49704253036648,20.1218000776565,2.16153189778506));
#4063=CARTESIAN_POINT('Ctrl Pts',(-1.98934597530643,20.2468000776565,1.51515420778634));
#4064=CARTESIAN_POINT('Ctrl Pts',(-2.48164942024637,20.3718000776565,0.868776517787626));
#4065=CARTESIAN_POINT('Ctrl Pts',(-2.5,20.4968000776565,0.0564772772053586));
#4066=CARTESIAN_POINT('Ctrl Pts',(-2.51835057975363,20.6218000776565,-0.755821963376908));
#4067=CARTESIAN_POINT('Ctrl Pts',(-2.05573899656831,20.7468000776565,-1.42377205367602));
#4068=CARTESIAN_POINT('Ctrl Pts',(-1.593127413383,20.8718000776565,-2.09172214397514));
#4069=CARTESIAN_POINT('Ctrl Pts',(-0.826255568446133,20.9968000776565,-2.3601888522854));
#4070=CARTESIAN_POINT('Ctrl Pts',(-0.0593837235092677,21.1218000776565,
-2.62865556059567));
#4071=CARTESIAN_POINT('Ctrl Pts',(0.718829403428605,21.2468000776565,-2.39509372919037));
#4072=CARTESIAN_POINT('Ctrl Pts',(1.49704253036648,21.3718000776565,-2.16153189778506));
#4073=CARTESIAN_POINT('Ctrl Pts',(1.98934597530643,21.4968000776565,-1.51515420778634));
#4074=CARTESIAN_POINT('Ctrl Pts',(2.48164942024637,21.6218000776565,-0.868776517787625));
#4075=CARTESIAN_POINT('Ctrl Pts',(2.5,21.7468000776565,-0.0564772772053589));
#4076=CARTESIAN_POINT('Ctrl Pts',(2.51835057975363,21.8718000776565,0.755821963376907));
#4077=CARTESIAN_POINT('Ctrl Pts',(2.05573899656831,21.9968000776565,1.42377205367602));
#4078=CARTESIAN_POINT('Ctrl Pts',(1.593127413383,22.1218000776565,2.09172214397514));
#4079=CARTESIAN_POINT('Ctrl Pts',(0.826255568446133,22.2468000776565,2.3601888522854));
#4080=CARTESIAN_POINT('Ctrl Pts',(0.059383723509268,22.3718000776565,2.62865556059567));
#4081=CARTESIAN_POINT('Ctrl Pts',(-0.718829403428604,22.4968000776565,2.39509372919037));
#4082=CARTESIAN_POINT('Ctrl Pts',(-1.49704253036648,22.6218000776565,2.16153189778506));
#4083=CARTESIAN_POINT('Ctrl Pts',(-1.98934597530643,22.7468000776565,1.51515420778634));
#4084=CARTESIAN_POINT('Ctrl Pts',(-2.48164942024637,22.8718000776565,0.868776517787626));
#4085=CARTESIAN_POINT('Ctrl Pts',(-2.5,22.9968000776565,0.0564772772053586));
#4086=CARTESIAN_POINT('Ctrl Pts',(-2.51835057975363,23.1218000776565,-0.755821963376908));
#4087=CARTESIAN_POINT('Ctrl Pts',(-2.05573899656831,23.2468000776565,-1.42377205367602));
#4088=CARTESIAN_POINT('Ctrl Pts',(-1.593127413383,23.3718000776565,-2.09172214397514));
#4089=CARTESIAN_POINT('Ctrl Pts',(-0.826255568446133,23.4968000776565,-2.3601888522854));
#4090=CARTESIAN_POINT('Ctrl Pts',(-0.0593837235092677,23.6218000776565,
-2.62865556059567));
#4091=CARTESIAN_POINT('Ctrl Pts',(0.718829403428605,23.7468000776565,-2.39509372919037));
#4092=CARTESIAN_POINT('Ctrl Pts',(1.49704253036648,23.8718000776565,-2.16153189778506));
#4093=CARTESIAN_POINT('Ctrl Pts',(1.98934597530643,23.9968000776565,-1.51515420778634));
#4094=CARTESIAN_POINT('Ctrl Pts',(2.48164942024637,24.1218000776565,-0.868776517787625));
#4095=CARTESIAN_POINT('Ctrl Pts',(2.5,24.2468000776565,-0.0564772772053589));
#4096=CARTESIAN_POINT('Ctrl Pts',(2.51835057975363,24.3718000776565,0.755821963376907));
#4097=CARTESIAN_POINT('Ctrl Pts',(2.05573899656831,24.4968000776565,1.42377205367602));
#4098=CARTESIAN_POINT('Ctrl Pts',(1.593127413383,24.6218000776565,2.09172214397514));
#4099=CARTESIAN_POINT('Ctrl Pts',(0.826255568446133,24.7468000776565,2.3601888522854));
#4100=CARTESIAN_POINT('Ctrl Pts',(0.059383723509268,24.8718000776565,2.62865556059567));
#4101=CARTESIAN_POINT('Ctrl Pts',(-0.718829403428604,24.9968000776565,2.39509372919037));
#4102=CARTESIAN_POINT('Ctrl Pts',(-1.49704253036648,25.1218000776565,2.16153189778506));
#4103=CARTESIAN_POINT('Ctrl Pts',(-1.98934597530643,25.2468000776565,1.51515420778634));
#4104=CARTESIAN_POINT('Ctrl Pts',(-2.48164942024637,25.3718000776565,0.868776517787626));
#4105=CARTESIAN_POINT('Ctrl Pts',(-2.5,25.4968000776565,0.0564772772053586));
#4106=CARTESIAN_POINT('Ctrl Pts',(-2.51835057975363,25.6218000776565,-0.755821963376908));
#4107=CARTESIAN_POINT('Ctrl Pts',(-2.05573899656831,25.7468000776565,-1.42377205367602));
#4108=CARTESIAN_POINT('Ctrl Pts',(-1.593127413383,25.8718000776565,-2.09172214397514));
#4109=CARTESIAN_POINT('Ctrl Pts',(-0.826255568446133,25.9968000776565,-2.3601888522854));
#4110=CARTESIAN_POINT('Ctrl Pts',(-0.0593837235092677,26.1218000776565,
-2.62865556059567));
#4111=CARTESIAN_POINT('Ctrl Pts',(0.718829403428605,26.2468000776565,-2.39509372919037));
#4112=CARTESIAN_POINT('Ctrl Pts',(1.49704253036648,26.3718000776565,-2.16153189778506));
#4113=CARTESIAN_POINT('Ctrl Pts',(1.98934597530643,26.4968000776565,-1.51515420778634));
#4114=CARTESIAN_POINT('Ctrl Pts',(2.48164942024637,26.6218000776565,-0.868776517787625));
#4115=CARTESIAN_POINT('Ctrl Pts',(2.5,26.7468000776565,-0.0564772772053589));
#4116=CARTESIAN_POINT('Ctrl Pts',(2.51835057975363,26.8718000776565,0.755821963376907));
#4117=CARTESIAN_POINT('Ctrl Pts',(2.05573899656831,26.9968000776565,1.42377205367602));
#4118=CARTESIAN_POINT('Ctrl Pts',(1.593127413383,27.1218000776565,2.09172214397514));
#4119=CARTESIAN_POINT('Ctrl Pts',(0.826255568446133,27.2468000776565,2.3601888522854));
#4120=CARTESIAN_POINT('Ctrl Pts',(0.059383723509268,27.3718000776565,2.62865556059567));
#4121=CARTESIAN_POINT('Ctrl Pts',(-0.718829403428604,27.4968000776565,2.39509372919037));
#4122=CARTESIAN_POINT('Ctrl Pts',(-1.49704253036648,27.6218000776565,2.16153189778506));
#4123=CARTESIAN_POINT('Ctrl Pts',(-1.98934597530643,27.7468000776565,1.51515420778634));
#4124=CARTESIAN_POINT('Ctrl Pts',(-2.48164942024637,27.8718000776565,0.868776517787626));
#4125=CARTESIAN_POINT('Ctrl Pts',(-2.5,27.9968000776565,0.0564772772053586));
#4126=CARTESIAN_POINT('Ctrl Pts',(-2.51835057975363,28.1218000776565,-0.755821963376908));
#4127=CARTESIAN_POINT('Ctrl Pts',(-2.05573899656831,28.2468000776565,-1.42377205367602));
#4128=CARTESIAN_POINT('Ctrl Pts',(-1.593127413383,28.3718000776565,-2.09172214397514));
#4129=CARTESIAN_POINT('Ctrl Pts',(-0.826255568446133,28.4968000776565,-2.3601888522854));
#4130=CARTESIAN_POINT('Ctrl Pts',(-0.0593837235092677,28.6218000776565,
-2.62865556059567));
#4131=CARTESIAN_POINT('Ctrl Pts',(0.718829403428605,28.7468000776565,-2.39509372919037));
#4132=CARTESIAN_POINT('Ctrl Pts',(1.49704253036648,28.8718000776565,-2.16153189778506));
#4133=CARTESIAN_POINT('Ctrl Pts',(1.98934597530643,28.9968000776565,-1.51515420778634));
#4134=CARTESIAN_POINT('Ctrl Pts',(2.48164942024637,29.1218000776565,-0.868776517787625));
#4135=CARTESIAN_POINT('Ctrl Pts',(2.5,29.2468000776565,-0.0564772772053589));
#4136=CARTESIAN_POINT('Ctrl Pts',(2.51835057975363,29.3718000776565,0.755821963376907));
#4137=CARTESIAN_POINT('Ctrl Pts',(2.05573899656831,29.4968000776565,1.42377205367602));
#4138=CARTESIAN_POINT('Ctrl Pts',(1.593127413383,29.6218000776565,2.09172214397514));
#4139=CARTESIAN_POINT('Ctrl Pts',(0.826255568446133,29.7468000776565,2.3601888522854));
#4140=CARTESIAN_POINT('Ctrl Pts',(0.059383723509268,29.8718000776565,2.62865556059567));
#4141=CARTESIAN_POINT('Ctrl Pts',(-0.718829403428604,29.9968000776565,2.39509372919037));
#4142=CARTESIAN_POINT('Ctrl Pts',(-1.49704253036648,30.1218000776565,2.16153189778506));
#4143=CARTESIAN_POINT('Ctrl Pts',(-1.98934597530643,30.2468000776565,1.51515420778634));
#4144=CARTESIAN_POINT('Ctrl Pts',(-2.48164942024637,30.3718000776565,0.868776517787626));
#4145=CARTESIAN_POINT('Ctrl Pts',(-2.5,30.4968000776565,0.0564772772053586));
#4146=CARTESIAN_POINT('Ctrl Pts',(-2.51835057975363,30.6218000776565,-0.755821963376908));
#4147=CARTESIAN_POINT('Ctrl Pts',(-2.05573899656831,30.7468000776565,-1.42377205367602));
#4148=CARTESIAN_POINT('Ctrl Pts',(-1.593127413383,30.8718000776565,-2.09172214397514));
#4149=CARTESIAN_POINT('Ctrl Pts',(-0.826255568446133,30.9968000776565,-2.3601888522854));
#4150=CARTESIAN_POINT('Ctrl Pts',(-0.0593837235092677,31.1218000776565,
-2.62865556059567));
#4151=CARTESIAN_POINT('Ctrl Pts',(0.718829403428605,31.2468000776565,-2.39509372919037));
#4152=CARTESIAN_POINT('Ctrl Pts',(1.49704253036648,31.3718000776565,-2.16153189778506));
#4153=CARTESIAN_POINT('Ctrl Pts',(1.98934597530643,31.4968000776565,-1.51515420778634));
#4154=CARTESIAN_POINT('Ctrl Pts',(2.48164942024637,31.6218000776565,-0.868776517787625));
#4155=CARTESIAN_POINT('Ctrl Pts',(2.5,31.7468000776565,-0.0564772772053589));
#4156=CARTESIAN_POINT('Ctrl Pts',(2.51835057975363,31.8718000776565,0.755821963376907));
#4157=CARTESIAN_POINT('Ctrl Pts',(2.05573899656831,31.9968000776565,1.42377205367602));
#4158=CARTESIAN_POINT('Ctrl Pts',(1.593127413383,32.1218000776565,2.09172214397514));
#4159=CARTESIAN_POINT('Ctrl Pts',(0.826255568446133,32.2468000776565,2.3601888522854));
#4160=CARTESIAN_POINT('Ctrl Pts',(0.059383723509268,32.3718000776565,2.62865556059567));
#4161=CARTESIAN_POINT('Ctrl Pts',(-0.718829403428604,32.4968000776565,2.39509372919037));
#4162=CARTESIAN_POINT('Ctrl Pts',(-1.49704253036648,32.6218000776565,2.16153189778506));
#4163=CARTESIAN_POINT('Ctrl Pts',(-1.98934597530643,32.7468000776565,1.51515420778634));
#4164=CARTESIAN_POINT('Ctrl Pts',(-2.48164942024637,32.8718000776565,0.868776517787626));
#4165=CARTESIAN_POINT('Ctrl Pts',(-2.5,32.9968000776565,0.0564772772053586));
#4166=CARTESIAN_POINT('Ctrl Pts',(-2.51835057975363,33.1218000776565,-0.755821963376908));
#4167=CARTESIAN_POINT('Ctrl Pts',(-2.05573899656831,33.2468000776565,-1.42377205367602));
#4168=CARTESIAN_POINT('Ctrl Pts',(-1.593127413383,33.3718000776565,-2.09172214397514));
#4169=CARTESIAN_POINT('Ctrl Pts',(-0.826255568446133,33.4968000776565,-2.3601888522854));
#4170=CARTESIAN_POINT('Ctrl Pts',(-0.0593837235092677,33.6218000776565,
-2.62865556059567));
#4171=CARTESIAN_POINT('Ctrl Pts',(0.718829403428605,33.7468000776565,-2.39509372919037));
#4172=CARTESIAN_POINT('Ctrl Pts',(1.49704253036648,33.8718000776565,-2.16153189778506));
#4173=CARTESIAN_POINT('Ctrl Pts',(1.98934597530643,33.9968000776565,-1.51515420778634));
#4174=CARTESIAN_POINT('Ctrl Pts',(2.48164942024637,34.1218000776565,-0.868776517787625));
#4175=CARTESIAN_POINT('Ctrl Pts',(2.5,34.2468000776565,-0.0564772772053589));
#4176=CARTESIAN_POINT('Ctrl Pts',(2.51835057975363,34.3718000776565,0.755821963376907));
#4177=CARTESIAN_POINT('Ctrl Pts',(2.05573899656831,34.4968000776565,1.42377205367602));
#4178=CARTESIAN_POINT('Ctrl Pts',(1.593127413383,34.6218000776565,2.09172214397514));
#4179=CARTESIAN_POINT('Ctrl Pts',(0.826255568446133,34.7468000776565,2.3601888522854));
#4180=CARTESIAN_POINT('Ctrl Pts',(0.059383723509268,34.8718000776565,2.62865556059567));
#4181=CARTESIAN_POINT('Ctrl Pts',(-0.718829403428604,34.9968000776565,2.39509372919037));
#4182=CARTESIAN_POINT('Ctrl Pts',(-1.49704253036648,35.1218000776565,2.16153189778506));
#4183=CARTESIAN_POINT('Ctrl Pts',(-1.98934597530643,35.2468000776565,1.51515420778634));
#4184=CARTESIAN_POINT('Ctrl Pts',(-2.48164942024637,35.3718000776565,0.868776517787626));
#4185=CARTESIAN_POINT('Ctrl Pts',(-2.5,35.4968000776565,0.0564772772053586));
#4186=CARTESIAN_POINT('Ctrl Pts',(-2.51835057975363,35.6218000776565,-0.755821963376908));
#4187=CARTESIAN_POINT('Ctrl Pts',(-2.05573899656831,35.7468000776565,-1.42377205367602));
#4188=CARTESIAN_POINT('Ctrl Pts',(-1.593127413383,35.8718000776565,-2.09172214397514));
#4189=CARTESIAN_POINT('Ctrl Pts',(-0.826255568446133,35.9968000776565,-2.3601888522854));
#4190=CARTESIAN_POINT('Ctrl Pts',(-0.0593837235092677,36.1218000776565,
-2.62865556059567));
#4191=CARTESIAN_POINT('Ctrl Pts',(0.718829403428605,36.2468000776565,-2.39509372919037));
#4192=CARTESIAN_POINT('Ctrl Pts',(1.49704253036648,36.3718000776565,-2.16153189778506));
#4193=CARTESIAN_POINT('Ctrl Pts',(1.98934597530643,36.4968000776565,-1.51515420778634));
#4194=CARTESIAN_POINT('Ctrl Pts',(2.48164942024637,36.6218000776565,-0.868776517787625));
#4195=CARTESIAN_POINT('Ctrl Pts',(2.5,36.7468000776565,-0.0564772772053589));
#4196=CARTESIAN_POINT('Ctrl Pts',(2.51835057975363,36.8718000776565,0.755821963376907));
#4197=CARTESIAN_POINT('Ctrl Pts',(2.05573899656831,36.9968000776565,1.42377205367602));
#4198=CARTESIAN_POINT('Ctrl Pts',(1.593127413383,37.1218000776565,2.09172214397514));
#4199=CARTESIAN_POINT('Ctrl Pts',(0.826255568446133,37.2468000776565,2.3601888522854));
#4200=CARTESIAN_POINT('Ctrl Pts',(0.059383723509268,37.3718000776565,2.62865556059567));
#4201=CARTESIAN_POINT('Ctrl Pts',(-0.718829403428604,37.4968000776565,2.39509372919037));
#4202=CARTESIAN_POINT('Ctrl Pts',(-1.49704253036648,37.6218000776565,2.16153189778506));
#4203=CARTESIAN_POINT('Ctrl Pts',(-1.98934597530643,37.7468000776565,1.51515420778634));
#4204=CARTESIAN_POINT('Ctrl Pts',(-2.48164942024637,37.8718000776565,0.868776517787626));
#4205=CARTESIAN_POINT('Ctrl Pts',(-2.5,37.9968000776565,0.0564772772053586));
#4206=CARTESIAN_POINT('Ctrl Pts',(-2.51835057975363,38.1218000776565,-0.755821963376908));
#4207=CARTESIAN_POINT('Ctrl Pts',(-2.05573899656831,38.2468000776565,-1.42377205367602));
#4208=CARTESIAN_POINT('Ctrl Pts',(-1.593127413383,38.3718000776565,-2.09172214397514));
#4209=CARTESIAN_POINT('Ctrl Pts',(-0.826255568446133,38.4968000776565,-2.3601888522854));
#4210=CARTESIAN_POINT('Ctrl Pts',(-0.0593837235092677,38.6218000776565,
-2.62865556059567));
#4211=CARTESIAN_POINT('Ctrl Pts',(0.718829403428605,38.7468000776565,-2.39509372919037));
#4212=CARTESIAN_POINT('Ctrl Pts',(1.49704253036648,38.8718000776565,-2.16153189778506));
#4213=CARTESIAN_POINT('Ctrl Pts',(1.98934597530643,38.9968000776565,-1.51515420778634));
#4214=CARTESIAN_POINT('Ctrl Pts',(2.48164942024637,39.1218000776565,-0.868776517787625));
#4215=CARTESIAN_POINT('Ctrl Pts',(2.5,39.2468000776565,-0.0564772772053589));
#4216=CARTESIAN_POINT('Ctrl Pts',(2.51835057975363,39.3718000776565,0.755821963376907));
#4217=CARTESIAN_POINT('Ctrl Pts',(2.05573899656831,39.4968000776565,1.42377205367602));
#4218=CARTESIAN_POINT('Ctrl Pts',(1.593127413383,39.6218000776565,2.09172214397514));
#4219=CARTESIAN_POINT('Ctrl Pts',(0.826255568446133,39.7468000776565,2.3601888522854));
#4220=CARTESIAN_POINT('Ctrl Pts',(0.059383723509268,39.8718000776565,2.62865556059567));
#4221=CARTESIAN_POINT('Ctrl Pts',(-0.718829403428604,39.9968000776565,2.39509372919037));
#4222=CARTESIAN_POINT('Ctrl Pts',(-1.49704253036648,40.1218000776565,2.16153189778506));
#4223=CARTESIAN_POINT('Ctrl Pts',(-1.98934597530643,40.2468000776565,1.51515420778634));
#4224=CARTESIAN_POINT('Ctrl Pts',(-2.48164942024637,40.3718000776565,0.868776517787626));
#4225=CARTESIAN_POINT('Ctrl Pts',(-2.5,40.4968000776565,0.0564772772053586));
#4226=CARTESIAN_POINT('Ctrl Pts',(-2.5,14.5031999223435,-0.056477277205306));
#4227=CARTESIAN_POINT('Ctrl Pts',(-2.48164942024639,14.6281999223435,-0.868776517787572));
#4228=CARTESIAN_POINT('Ctrl Pts',(-1.98934597530646,14.7531999223435,-1.5151542077863));
#4229=CARTESIAN_POINT('Ctrl Pts',(-1.49704253036652,14.8781999223435,-2.16153189778503));
#4230=CARTESIAN_POINT('Ctrl Pts',(-0.718829403428655,15.0031999223435,-2.39509372919035));
#4231=CARTESIAN_POINT('Ctrl Pts',(0.0593837235092121,15.1281999223435,-2.62865556059567));
#4232=CARTESIAN_POINT('Ctrl Pts',(0.826255568446083,15.2531999223435,-2.36018885228542));
#4233=CARTESIAN_POINT('Ctrl Pts',(1.59312741338295,15.3781999223435,-2.09172214397517));
#4234=CARTESIAN_POINT('Ctrl Pts',(2.05573899656828,15.5031999223436,-1.42377205367607));
#4235=CARTESIAN_POINT('Ctrl Pts',(2.51835057975361,15.6281999223435,-0.755821963376961));
#4236=CARTESIAN_POINT('Ctrl Pts',(2.5,15.7531999223435,0.0564772772053057));
#4237=CARTESIAN_POINT('Ctrl Pts',(2.48164942024639,15.8781999223435,0.868776517787572));
#4238=CARTESIAN_POINT('Ctrl Pts',(1.98934597530646,16.0031999223435,1.5151542077863));
#4239=CARTESIAN_POINT('Ctrl Pts',(1.49704253036652,16.1281999223435,2.16153189778503));
#4240=CARTESIAN_POINT('Ctrl Pts',(0.718829403428655,16.2531999223435,2.39509372919035));
#4241=CARTESIAN_POINT('Ctrl Pts',(-0.0593837235092117,16.3781999223435,
2.62865556059567));
#4242=CARTESIAN_POINT('Ctrl Pts',(-0.826255568446083,16.5031999223435,2.36018885228542));
#4243=CARTESIAN_POINT('Ctrl Pts',(-1.59312741338295,16.6281999223435,2.09172214397517));
#4244=CARTESIAN_POINT('Ctrl Pts',(-2.05573899656828,16.7531999223435,1.42377205367607));
#4245=CARTESIAN_POINT('Ctrl Pts',(-2.51835057975361,16.8781999223435,0.755821963376961));
#4246=CARTESIAN_POINT('Ctrl Pts',(-2.5,17.0031999223435,-0.056477277205306));
#4247=CARTESIAN_POINT('Ctrl Pts',(-2.48164942024639,17.1281999223435,-0.868776517787572));
#4248=CARTESIAN_POINT('Ctrl Pts',(-1.98934597530646,17.2531999223435,-1.5151542077863));
#4249=CARTESIAN_POINT('Ctrl Pts',(-1.49704253036652,17.3781999223435,-2.16153189778503));
#4250=CARTESIAN_POINT('Ctrl Pts',(-0.718829403428655,17.5031999223435,-2.39509372919035));
#4251=CARTESIAN_POINT('Ctrl Pts',(0.0593837235092121,17.6281999223435,-2.62865556059567));
#4252=CARTESIAN_POINT('Ctrl Pts',(0.826255568446083,17.7531999223435,-2.36018885228542));
#4253=CARTESIAN_POINT('Ctrl Pts',(1.59312741338295,17.8781999223435,-2.09172214397517));
#4254=CARTESIAN_POINT('Ctrl Pts',(2.05573899656828,18.0031999223435,-1.42377205367607));
#4255=CARTESIAN_POINT('Ctrl Pts',(2.51835057975361,18.1281999223435,-0.755821963376961));
#4256=CARTESIAN_POINT('Ctrl Pts',(2.5,18.2531999223435,0.0564772772053057));
#4257=CARTESIAN_POINT('Ctrl Pts',(2.48164942024639,18.3781999223435,0.868776517787572));
#4258=CARTESIAN_POINT('Ctrl Pts',(1.98934597530646,18.5031999223435,1.5151542077863));
#4259=CARTESIAN_POINT('Ctrl Pts',(1.49704253036652,18.6281999223435,2.16153189778503));
#4260=CARTESIAN_POINT('Ctrl Pts',(0.718829403428655,18.7531999223435,2.39509372919035));
#4261=CARTESIAN_POINT('Ctrl Pts',(-0.0593837235092117,18.8781999223435,
2.62865556059567));
#4262=CARTESIAN_POINT('Ctrl Pts',(-0.826255568446083,19.0031999223435,2.36018885228542));
#4263=CARTESIAN_POINT('Ctrl Pts',(-1.59312741338295,19.1281999223435,2.09172214397517));
#4264=CARTESIAN_POINT('Ctrl Pts',(-2.05573899656828,19.2531999223435,1.42377205367607));
#4265=CARTESIAN_POINT('Ctrl Pts',(-2.51835057975361,19.3781999223435,0.755821963376961));
#4266=CARTESIAN_POINT('Ctrl Pts',(-2.5,19.5031999223435,-0.056477277205306));
#4267=CARTESIAN_POINT('Ctrl Pts',(-2.48164942024639,19.6281999223435,-0.868776517787572));
#4268=CARTESIAN_POINT('Ctrl Pts',(-1.98934597530646,19.7531999223435,-1.5151542077863));
#4269=CARTESIAN_POINT('Ctrl Pts',(-1.49704253036652,19.8781999223435,-2.16153189778503));
#4270=CARTESIAN_POINT('Ctrl Pts',(-0.718829403428655,20.0031999223435,-2.39509372919035));
#4271=CARTESIAN_POINT('Ctrl Pts',(0.0593837235092121,20.1281999223436,-2.62865556059567));
#4272=CARTESIAN_POINT('Ctrl Pts',(0.826255568446083,20.2531999223435,-2.36018885228542));
#4273=CARTESIAN_POINT('Ctrl Pts',(1.59312741338295,20.3781999223435,-2.09172214397517));
#4274=CARTESIAN_POINT('Ctrl Pts',(2.05573899656828,20.5031999223436,-1.42377205367607));
#4275=CARTESIAN_POINT('Ctrl Pts',(2.51835057975361,20.6281999223435,-0.755821963376961));
#4276=CARTESIAN_POINT('Ctrl Pts',(2.5,20.7531999223436,0.0564772772053057));
#4277=CARTESIAN_POINT('Ctrl Pts',(2.48164942024639,20.8781999223436,0.868776517787572));
#4278=CARTESIAN_POINT('Ctrl Pts',(1.98934597530646,21.0031999223435,1.5151542077863));
#4279=CARTESIAN_POINT('Ctrl Pts',(1.49704253036652,21.1281999223435,2.16153189778503));
#4280=CARTESIAN_POINT('Ctrl Pts',(0.718829403428655,21.2531999223435,2.39509372919035));
#4281=CARTESIAN_POINT('Ctrl Pts',(-0.0593837235092117,21.3781999223435,
2.62865556059567));
#4282=CARTESIAN_POINT('Ctrl Pts',(-0.826255568446083,21.5031999223435,2.36018885228542));
#4283=CARTESIAN_POINT('Ctrl Pts',(-1.59312741338295,21.6281999223435,2.09172214397517));
#4284=CARTESIAN_POINT('Ctrl Pts',(-2.05573899656828,21.7531999223435,1.42377205367607));
#4285=CARTESIAN_POINT('Ctrl Pts',(-2.51835057975361,21.8781999223435,0.755821963376961));
#4286=CARTESIAN_POINT('Ctrl Pts',(-2.5,22.0031999223436,-0.056477277205306));
#4287=CARTESIAN_POINT('Ctrl Pts',(-2.48164942024639,22.1281999223435,-0.868776517787572));
#4288=CARTESIAN_POINT('Ctrl Pts',(-1.98934597530646,22.2531999223435,-1.5151542077863));
#4289=CARTESIAN_POINT('Ctrl Pts',(-1.49704253036652,22.3781999223435,-2.16153189778503));
#4290=CARTESIAN_POINT('Ctrl Pts',(-0.718829403428655,22.5031999223435,-2.39509372919035));
#4291=CARTESIAN_POINT('Ctrl Pts',(0.0593837235092121,22.6281999223436,-2.62865556059567));
#4292=CARTESIAN_POINT('Ctrl Pts',(0.826255568446083,22.7531999223435,-2.36018885228542));
#4293=CARTESIAN_POINT('Ctrl Pts',(1.59312741338295,22.8781999223435,-2.09172214397517));
#4294=CARTESIAN_POINT('Ctrl Pts',(2.05573899656828,23.0031999223435,-1.42377205367607));
#4295=CARTESIAN_POINT('Ctrl Pts',(2.51835057975361,23.1281999223435,-0.755821963376961));
#4296=CARTESIAN_POINT('Ctrl Pts',(2.5,23.2531999223436,0.0564772772053057));
#4297=CARTESIAN_POINT('Ctrl Pts',(2.48164942024639,23.3781999223435,0.868776517787572));
#4298=CARTESIAN_POINT('Ctrl Pts',(1.98934597530646,23.5031999223436,1.5151542077863));
#4299=CARTESIAN_POINT('Ctrl Pts',(1.49704253036652,23.6281999223435,2.16153189778503));
#4300=CARTESIAN_POINT('Ctrl Pts',(0.718829403428655,23.7531999223435,2.39509372919035));
#4301=CARTESIAN_POINT('Ctrl Pts',(-0.0593837235092117,23.8781999223435,
2.62865556059567));
#4302=CARTESIAN_POINT('Ctrl Pts',(-0.826255568446083,24.0031999223435,2.36018885228542));
#4303=CARTESIAN_POINT('Ctrl Pts',(-1.59312741338295,24.1281999223435,2.09172214397517));
#4304=CARTESIAN_POINT('Ctrl Pts',(-2.05573899656828,24.2531999223435,1.42377205367607));
#4305=CARTESIAN_POINT('Ctrl Pts',(-2.51835057975361,24.3781999223435,0.755821963376961));
#4306=CARTESIAN_POINT('Ctrl Pts',(-2.5,24.5031999223436,-0.056477277205306));
#4307=CARTESIAN_POINT('Ctrl Pts',(-2.48164942024639,24.6281999223435,-0.868776517787572));
#4308=CARTESIAN_POINT('Ctrl Pts',(-1.98934597530646,24.7531999223435,-1.5151542077863));
#4309=CARTESIAN_POINT('Ctrl Pts',(-1.49704253036652,24.8781999223436,-2.16153189778503));
#4310=CARTESIAN_POINT('Ctrl Pts',(-0.718829403428655,25.0031999223435,-2.39509372919035));
#4311=CARTESIAN_POINT('Ctrl Pts',(0.0593837235092121,25.1281999223435,-2.62865556059567));
#4312=CARTESIAN_POINT('Ctrl Pts',(0.826255568446083,25.2531999223435,-2.36018885228542));
#4313=CARTESIAN_POINT('Ctrl Pts',(1.59312741338295,25.3781999223435,-2.09172214397517));
#4314=CARTESIAN_POINT('Ctrl Pts',(2.05573899656828,25.5031999223435,-1.42377205367607));
#4315=CARTESIAN_POINT('Ctrl Pts',(2.51835057975361,25.6281999223435,-0.755821963376961));
#4316=CARTESIAN_POINT('Ctrl Pts',(2.5,25.7531999223436,0.0564772772053057));
#4317=CARTESIAN_POINT('Ctrl Pts',(2.48164942024639,25.8781999223436,0.868776517787572));
#4318=CARTESIAN_POINT('Ctrl Pts',(1.98934597530646,26.0031999223435,1.5151542077863));
#4319=CARTESIAN_POINT('Ctrl Pts',(1.49704253036652,26.1281999223435,2.16153189778503));
#4320=CARTESIAN_POINT('Ctrl Pts',(0.718829403428655,26.2531999223435,2.39509372919035));
#4321=CARTESIAN_POINT('Ctrl Pts',(-0.0593837235092117,26.3781999223436,
2.62865556059567));
#4322=CARTESIAN_POINT('Ctrl Pts',(-0.826255568446083,26.5031999223435,2.36018885228542));
#4323=CARTESIAN_POINT('Ctrl Pts',(-1.59312741338295,26.6281999223435,2.09172214397517));
#4324=CARTESIAN_POINT('Ctrl Pts',(-2.05573899656828,26.7531999223436,1.42377205367607));
#4325=CARTESIAN_POINT('Ctrl Pts',(-2.51835057975361,26.8781999223435,0.755821963376961));
#4326=CARTESIAN_POINT('Ctrl Pts',(-2.5,27.0031999223436,-0.056477277205306));
#4327=CARTESIAN_POINT('Ctrl Pts',(-2.48164942024639,27.1281999223436,-0.868776517787572));
#4328=CARTESIAN_POINT('Ctrl Pts',(-1.98934597530646,27.2531999223435,-1.5151542077863));
#4329=CARTESIAN_POINT('Ctrl Pts',(-1.49704253036652,27.3781999223436,-2.16153189778503));
#4330=CARTESIAN_POINT('Ctrl Pts',(-0.718829403428655,27.5031999223435,-2.39509372919035));
#4331=CARTESIAN_POINT('Ctrl Pts',(0.0593837235092121,27.6281999223435,-2.62865556059567));
#4332=CARTESIAN_POINT('Ctrl Pts',(0.826255568446083,27.7531999223436,-2.36018885228542));
#4333=CARTESIAN_POINT('Ctrl Pts',(1.59312741338295,27.8781999223436,-2.09172214397517));
#4334=CARTESIAN_POINT('Ctrl Pts',(2.05573899656828,28.0031999223436,-1.42377205367607));
#4335=CARTESIAN_POINT('Ctrl Pts',(2.51835057975361,28.1281999223436,-0.755821963376961));
#4336=CARTESIAN_POINT('Ctrl Pts',(2.5,28.2531999223436,0.0564772772053057));
#4337=CARTESIAN_POINT('Ctrl Pts',(2.48164942024639,28.3781999223436,0.868776517787572));
#4338=CARTESIAN_POINT('Ctrl Pts',(1.98934597530646,28.5031999223436,1.5151542077863));
#4339=CARTESIAN_POINT('Ctrl Pts',(1.49704253036652,28.6281999223436,2.16153189778503));
#4340=CARTESIAN_POINT('Ctrl Pts',(0.718829403428655,28.7531999223435,2.39509372919035));
#4341=CARTESIAN_POINT('Ctrl Pts',(-0.0593837235092117,28.8781999223435,
2.62865556059567));
#4342=CARTESIAN_POINT('Ctrl Pts',(-0.826255568446083,29.0031999223436,2.36018885228542));
#4343=CARTESIAN_POINT('Ctrl Pts',(-1.59312741338295,29.1281999223435,2.09172214397517));
#4344=CARTESIAN_POINT('Ctrl Pts',(-2.05573899656828,29.2531999223436,1.42377205367607));
#4345=CARTESIAN_POINT('Ctrl Pts',(-2.51835057975361,29.3781999223436,0.755821963376961));
#4346=CARTESIAN_POINT('Ctrl Pts',(-2.5,29.5031999223436,-0.056477277205306));
#4347=CARTESIAN_POINT('Ctrl Pts',(-2.48164942024639,29.6281999223435,-0.868776517787572));
#4348=CARTESIAN_POINT('Ctrl Pts',(-1.98934597530646,29.7531999223435,-1.5151542077863));
#4349=CARTESIAN_POINT('Ctrl Pts',(-1.49704253036652,29.8781999223435,-2.16153189778503));
#4350=CARTESIAN_POINT('Ctrl Pts',(-0.718829403428655,30.0031999223435,-2.39509372919035));
#4351=CARTESIAN_POINT('Ctrl Pts',(0.0593837235092121,30.1281999223435,-2.62865556059567));
#4352=CARTESIAN_POINT('Ctrl Pts',(0.826255568446083,30.2531999223435,-2.36018885228542));
#4353=CARTESIAN_POINT('Ctrl Pts',(1.59312741338295,30.3781999223435,-2.09172214397517));
#4354=CARTESIAN_POINT('Ctrl Pts',(2.05573899656828,30.5031999223436,-1.42377205367607));
#4355=CARTESIAN_POINT('Ctrl Pts',(2.51835057975361,30.6281999223436,-0.755821963376961));
#4356=CARTESIAN_POINT('Ctrl Pts',(2.5,30.7531999223435,0.0564772772053057));
#4357=CARTESIAN_POINT('Ctrl Pts',(2.48164942024639,30.8781999223435,0.868776517787572));
#4358=CARTESIAN_POINT('Ctrl Pts',(1.98934597530646,31.0031999223436,1.5151542077863));
#4359=CARTESIAN_POINT('Ctrl Pts',(1.49704253036652,31.1281999223435,2.16153189778503));
#4360=CARTESIAN_POINT('Ctrl Pts',(0.718829403428655,31.2531999223435,2.39509372919035));
#4361=CARTESIAN_POINT('Ctrl Pts',(-0.0593837235092117,31.3781999223435,
2.62865556059567));
#4362=CARTESIAN_POINT('Ctrl Pts',(-0.826255568446083,31.5031999223435,2.36018885228542));
#4363=CARTESIAN_POINT('Ctrl Pts',(-1.59312741338295,31.6281999223435,2.09172214397517));
#4364=CARTESIAN_POINT('Ctrl Pts',(-2.05573899656828,31.7531999223436,1.42377205367607));
#4365=CARTESIAN_POINT('Ctrl Pts',(-2.51835057975361,31.8781999223435,0.755821963376961));
#4366=CARTESIAN_POINT('Ctrl Pts',(-2.5,32.0031999223435,-0.056477277205306));
#4367=CARTESIAN_POINT('Ctrl Pts',(-2.48164942024639,32.1281999223435,-0.868776517787572));
#4368=CARTESIAN_POINT('Ctrl Pts',(-1.98934597530646,32.2531999223435,-1.5151542077863));
#4369=CARTESIAN_POINT('Ctrl Pts',(-1.49704253036652,32.3781999223435,-2.16153189778503));
#4370=CARTESIAN_POINT('Ctrl Pts',(-0.718829403428655,32.5031999223435,-2.39509372919035));
#4371=CARTESIAN_POINT('Ctrl Pts',(0.0593837235092121,32.6281999223435,-2.62865556059567));
#4372=CARTESIAN_POINT('Ctrl Pts',(0.826255568446083,32.7531999223435,-2.36018885228542));
#4373=CARTESIAN_POINT('Ctrl Pts',(1.59312741338295,32.8781999223435,-2.09172214397517));
#4374=CARTESIAN_POINT('Ctrl Pts',(2.05573899656828,33.0031999223436,-1.42377205367607));
#4375=CARTESIAN_POINT('Ctrl Pts',(2.51835057975361,33.1281999223435,-0.755821963376961));
#4376=CARTESIAN_POINT('Ctrl Pts',(2.5,33.2531999223435,0.0564772772053057));
#4377=CARTESIAN_POINT('Ctrl Pts',(2.48164942024639,33.3781999223435,0.868776517787572));
#4378=CARTESIAN_POINT('Ctrl Pts',(1.98934597530646,33.5031999223435,1.5151542077863));
#4379=CARTESIAN_POINT('Ctrl Pts',(1.49704253036652,33.6281999223436,2.16153189778503));
#4380=CARTESIAN_POINT('Ctrl Pts',(0.718829403428655,33.7531999223435,2.39509372919035));
#4381=CARTESIAN_POINT('Ctrl Pts',(-0.0593837235092117,33.8781999223435,
2.62865556059567));
#4382=CARTESIAN_POINT('Ctrl Pts',(-0.826255568446083,34.0031999223435,2.36018885228542));
#4383=CARTESIAN_POINT('Ctrl Pts',(-1.59312741338295,34.1281999223435,2.09172214397517));
#4384=CARTESIAN_POINT('Ctrl Pts',(-2.05573899656828,34.2531999223435,1.42377205367607));
#4385=CARTESIAN_POINT('Ctrl Pts',(-2.51835057975361,34.3781999223435,0.755821963376961));
#4386=CARTESIAN_POINT('Ctrl Pts',(-2.5,34.5031999223435,-0.056477277205306));
#4387=CARTESIAN_POINT('Ctrl Pts',(-2.48164942024639,34.6281999223435,-0.868776517787572));
#4388=CARTESIAN_POINT('Ctrl Pts',(-1.98934597530646,34.7531999223435,-1.5151542077863));
#4389=CARTESIAN_POINT('Ctrl Pts',(-1.49704253036652,34.8781999223436,-2.16153189778503));
#4390=CARTESIAN_POINT('Ctrl Pts',(-0.718829403428655,35.0031999223435,-2.39509372919035));
#4391=CARTESIAN_POINT('Ctrl Pts',(0.0593837235092121,35.1281999223435,-2.62865556059567));
#4392=CARTESIAN_POINT('Ctrl Pts',(0.826255568446083,35.2531999223435,-2.36018885228542));
#4393=CARTESIAN_POINT('Ctrl Pts',(1.59312741338295,35.3781999223435,-2.09172214397517));
#4394=CARTESIAN_POINT('Ctrl Pts',(2.05573899656828,35.5031999223436,-1.42377205367607));
#4395=CARTESIAN_POINT('Ctrl Pts',(2.51835057975361,35.6281999223435,-0.755821963376961));
#4396=CARTESIAN_POINT('Ctrl Pts',(2.5,35.7531999223435,0.0564772772053057));
#4397=CARTESIAN_POINT('Ctrl Pts',(2.48164942024639,35.8781999223435,0.868776517787572));
#4398=CARTESIAN_POINT('Ctrl Pts',(1.98934597530646,36.0031999223435,1.5151542077863));
#4399=CARTESIAN_POINT('Ctrl Pts',(1.49704253036652,36.1281999223436,2.16153189778503));
#4400=CARTESIAN_POINT('Ctrl Pts',(0.718829403428655,36.2531999223435,2.39509372919035));
#4401=CARTESIAN_POINT('Ctrl Pts',(-0.0593837235092117,36.3781999223435,
2.62865556059567));
#4402=CARTESIAN_POINT('Ctrl Pts',(-0.826255568446083,36.5031999223435,2.36018885228542));
#4403=CARTESIAN_POINT('Ctrl Pts',(-1.59312741338295,36.6281999223435,2.09172214397517));
#4404=CARTESIAN_POINT('Ctrl Pts',(-2.05573899656828,36.7531999223436,1.42377205367607));
#4405=CARTESIAN_POINT('Ctrl Pts',(-2.51835057975361,36.8781999223435,0.755821963376961));
#4406=CARTESIAN_POINT('Ctrl Pts',(-2.5,37.0031999223435,-0.056477277205306));
#4407=CARTESIAN_POINT('Ctrl Pts',(-2.48164942024639,37.1281999223435,-0.868776517787572));
#4408=CARTESIAN_POINT('Ctrl Pts',(-1.98934597530646,37.2531999223435,-1.5151542077863));
#4409=CARTESIAN_POINT('Ctrl Pts',(-1.49704253036652,37.3781999223436,-2.16153189778503));
#4410=CARTESIAN_POINT('Ctrl Pts',(-0.718829403428655,37.5031999223435,-2.39509372919035));
#4411=CARTESIAN_POINT('Ctrl Pts',(0.0593837235092121,37.6281999223435,-2.62865556059567));
#4412=CARTESIAN_POINT('Ctrl Pts',(0.826255568446083,37.7531999223435,-2.36018885228542));
#4413=CARTESIAN_POINT('Ctrl Pts',(1.59312741338295,37.8781999223435,-2.09172214397517));
#4414=CARTESIAN_POINT('Ctrl Pts',(2.05573899656828,38.0031999223435,-1.42377205367607));
#4415=CARTESIAN_POINT('Ctrl Pts',(2.51835057975361,38.1281999223435,-0.755821963376961));
#4416=CARTESIAN_POINT('Ctrl Pts',(2.5,38.2531999223435,0.0564772772053057));
#4417=CARTESIAN_POINT('Ctrl Pts',(2.48164942024639,38.3781999223435,0.868776517787572));
#4418=CARTESIAN_POINT('Ctrl Pts',(1.98934597530646,38.5031999223435,1.5151542077863));
#4419=CARTESIAN_POINT('Ctrl Pts',(1.49704253036652,38.6281999223436,2.16153189778503));
#4420=CARTESIAN_POINT('Ctrl Pts',(0.718829403428655,38.7531999223435,2.39509372919035));
#4421=CARTESIAN_POINT('Ctrl Pts',(-0.0593837235092117,38.8781999223435,
2.62865556059567));
#4422=CARTESIAN_POINT('Ctrl Pts',(-0.826255568446083,39.0031999223436,2.36018885228542));
#4423=CARTESIAN_POINT('Ctrl Pts',(-1.59312741338295,39.1281999223435,2.09172214397517));
#4424=CARTESIAN_POINT('Ctrl Pts',(-2.05573899656828,39.2531999223436,1.42377205367607));
#4425=CARTESIAN_POINT('Ctrl Pts',(-2.51835057975361,39.3781999223435,0.755821963376961));
#4426=CARTESIAN_POINT('Ctrl Pts',(-2.5,39.5031999223436,-0.056477277205306));
#4427=CARTESIAN_POINT('Ctrl Pts',(-3.5,14.5031999223435,-0.0564772772052956));
#4428=CARTESIAN_POINT('Ctrl Pts',(-3.48164942024639,14.6281999223435,-1.19369621402047));
#4429=CARTESIAN_POINT('Ctrl Pts',(-2.79836296968141,14.7531999223435,-2.10293946007877));
#4430=CARTESIAN_POINT('Ctrl Pts',(-2.11507651911643,14.8781999223435,-3.01218270613706));
#4431=CARTESIAN_POINT('Ctrl Pts',(-1.02784639780361,15.0031999223435,-3.3461502454855));
#4432=CARTESIAN_POINT('Ctrl Pts',(0.0593837235092011,15.1281999223435,-3.68011778483394));
#4433=CARTESIAN_POINT('Ctrl Pts',(1.13527256282102,15.2531999223435,-3.31124536858058));
#4434=CARTESIAN_POINT('Ctrl Pts',(2.21116140213284,15.3781999223435,-2.94237295232722));
#4435=CARTESIAN_POINT('Ctrl Pts',(2.86475599094322,15.5031999223435,-2.01155730596855));
#4436=CARTESIAN_POINT('Ctrl Pts',(3.51835057975361,15.6281999223435,-1.08074165960988));
#4437=CARTESIAN_POINT('Ctrl Pts',(3.5,15.7531999223435,0.0564772772052952));
#4438=CARTESIAN_POINT('Ctrl Pts',(3.48164942024639,15.8781999223435,1.19369621402047));
#4439=CARTESIAN_POINT('Ctrl Pts',(2.79836296968141,16.0031999223435,2.10293946007876));
#4440=CARTESIAN_POINT('Ctrl Pts',(2.11507651911643,16.1281999223435,3.01218270613706));
#4441=CARTESIAN_POINT('Ctrl Pts',(1.02784639780361,16.2531999223435,3.3461502454855));
#4442=CARTESIAN_POINT('Ctrl Pts',(-0.0593837235092006,16.3781999223435,
3.68011778483394));
#4443=CARTESIAN_POINT('Ctrl Pts',(-1.13527256282102,16.5031999223435,3.31124536858058));
#4444=CARTESIAN_POINT('Ctrl Pts',(-2.21116140213284,16.6281999223435,2.94237295232722));
#4445=CARTESIAN_POINT('Ctrl Pts',(-2.86475599094322,16.7531999223435,2.01155730596855));
#4446=CARTESIAN_POINT('Ctrl Pts',(-3.51835057975361,16.8781999223435,1.08074165960988));
#4447=CARTESIAN_POINT('Ctrl Pts',(-3.5,17.0031999223435,-0.0564772772052956));
#4448=CARTESIAN_POINT('Ctrl Pts',(-3.48164942024639,17.1281999223435,-1.19369621402047));
#4449=CARTESIAN_POINT('Ctrl Pts',(-2.79836296968141,17.2531999223435,-2.10293946007877));
#4450=CARTESIAN_POINT('Ctrl Pts',(-2.11507651911643,17.3781999223435,-3.01218270613706));
#4451=CARTESIAN_POINT('Ctrl Pts',(-1.02784639780361,17.5031999223435,-3.3461502454855));
#4452=CARTESIAN_POINT('Ctrl Pts',(0.0593837235092011,17.6281999223435,-3.68011778483394));
#4453=CARTESIAN_POINT('Ctrl Pts',(1.13527256282102,17.7531999223435,-3.31124536858058));
#4454=CARTESIAN_POINT('Ctrl Pts',(2.21116140213284,17.8781999223435,-2.94237295232722));
#4455=CARTESIAN_POINT('Ctrl Pts',(2.86475599094322,18.0031999223435,-2.01155730596855));
#4456=CARTESIAN_POINT('Ctrl Pts',(3.51835057975361,18.1281999223435,-1.08074165960988));
#4457=CARTESIAN_POINT('Ctrl Pts',(3.5,18.2531999223435,0.0564772772052952));
#4458=CARTESIAN_POINT('Ctrl Pts',(3.48164942024639,18.3781999223435,1.19369621402047));
#4459=CARTESIAN_POINT('Ctrl Pts',(2.79836296968141,18.5031999223435,2.10293946007876));
#4460=CARTESIAN_POINT('Ctrl Pts',(2.11507651911643,18.6281999223435,3.01218270613706));
#4461=CARTESIAN_POINT('Ctrl Pts',(1.02784639780361,18.7531999223435,3.3461502454855));
#4462=CARTESIAN_POINT('Ctrl Pts',(-0.0593837235092006,18.8781999223435,
3.68011778483394));
#4463=CARTESIAN_POINT('Ctrl Pts',(-1.13527256282102,19.0031999223435,3.31124536858058));
#4464=CARTESIAN_POINT('Ctrl Pts',(-2.21116140213284,19.1281999223435,2.94237295232722));
#4465=CARTESIAN_POINT('Ctrl Pts',(-2.86475599094322,19.2531999223435,2.01155730596855));
#4466=CARTESIAN_POINT('Ctrl Pts',(-3.51835057975361,19.3781999223435,1.08074165960988));
#4467=CARTESIAN_POINT('Ctrl Pts',(-3.5,19.5031999223435,-0.0564772772052956));
#4468=CARTESIAN_POINT('Ctrl Pts',(-3.48164942024639,19.6281999223435,-1.19369621402047));
#4469=CARTESIAN_POINT('Ctrl Pts',(-2.79836296968141,19.7531999223435,-2.10293946007877));
#4470=CARTESIAN_POINT('Ctrl Pts',(-2.11507651911643,19.8781999223435,-3.01218270613706));
#4471=CARTESIAN_POINT('Ctrl Pts',(-1.02784639780361,20.0031999223435,-3.3461502454855));
#4472=CARTESIAN_POINT('Ctrl Pts',(0.0593837235092011,20.1281999223435,-3.68011778483394));
#4473=CARTESIAN_POINT('Ctrl Pts',(1.13527256282102,20.2531999223435,-3.31124536858058));
#4474=CARTESIAN_POINT('Ctrl Pts',(2.21116140213284,20.3781999223435,-2.94237295232722));
#4475=CARTESIAN_POINT('Ctrl Pts',(2.86475599094322,20.5031999223435,-2.01155730596855));
#4476=CARTESIAN_POINT('Ctrl Pts',(3.51835057975361,20.6281999223435,-1.08074165960988));
#4477=CARTESIAN_POINT('Ctrl Pts',(3.5,20.7531999223435,0.0564772772052952));
#4478=CARTESIAN_POINT('Ctrl Pts',(3.48164942024639,20.8781999223435,1.19369621402047));
#4479=CARTESIAN_POINT('Ctrl Pts',(2.79836296968141,21.0031999223435,2.10293946007876));
#4480=CARTESIAN_POINT('Ctrl Pts',(2.11507651911643,21.1281999223435,3.01218270613706));
#4481=CARTESIAN_POINT('Ctrl Pts',(1.02784639780361,21.2531999223435,3.3461502454855));
#4482=CARTESIAN_POINT('Ctrl Pts',(-0.0593837235092006,21.3781999223435,
3.68011778483394));
#4483=CARTESIAN_POINT('Ctrl Pts',(-1.13527256282102,21.5031999223435,3.31124536858058));
#4484=CARTESIAN_POINT('Ctrl Pts',(-2.21116140213284,21.6281999223435,2.94237295232722));
#4485=CARTESIAN_POINT('Ctrl Pts',(-2.86475599094322,21.7531999223435,2.01155730596855));
#4486=CARTESIAN_POINT('Ctrl Pts',(-3.51835057975361,21.8781999223435,1.08074165960988));
#4487=CARTESIAN_POINT('Ctrl Pts',(-3.5,22.0031999223435,-0.0564772772052956));
#4488=CARTESIAN_POINT('Ctrl Pts',(-3.48164942024639,22.1281999223435,-1.19369621402047));
#4489=CARTESIAN_POINT('Ctrl Pts',(-2.79836296968141,22.2531999223435,-2.10293946007877));
#4490=CARTESIAN_POINT('Ctrl Pts',(-2.11507651911643,22.3781999223435,-3.01218270613706));
#4491=CARTESIAN_POINT('Ctrl Pts',(-1.02784639780361,22.5031999223435,-3.3461502454855));
#4492=CARTESIAN_POINT('Ctrl Pts',(0.0593837235092011,22.6281999223435,-3.68011778483394));
#4493=CARTESIAN_POINT('Ctrl Pts',(1.13527256282102,22.7531999223435,-3.31124536858058));
#4494=CARTESIAN_POINT('Ctrl Pts',(2.21116140213284,22.8781999223435,-2.94237295232722));
#4495=CARTESIAN_POINT('Ctrl Pts',(2.86475599094322,23.0031999223435,-2.01155730596855));
#4496=CARTESIAN_POINT('Ctrl Pts',(3.51835057975361,23.1281999223435,-1.08074165960988));
#4497=CARTESIAN_POINT('Ctrl Pts',(3.5,23.2531999223435,0.0564772772052952));
#4498=CARTESIAN_POINT('Ctrl Pts',(3.48164942024639,23.3781999223435,1.19369621402047));
#4499=CARTESIAN_POINT('Ctrl Pts',(2.79836296968141,23.5031999223435,2.10293946007876));
#4500=CARTESIAN_POINT('Ctrl Pts',(2.11507651911643,23.6281999223435,3.01218270613706));
#4501=CARTESIAN_POINT('Ctrl Pts',(1.02784639780361,23.7531999223435,3.3461502454855));
#4502=CARTESIAN_POINT('Ctrl Pts',(-0.0593837235092006,23.8781999223435,
3.68011778483394));
#4503=CARTESIAN_POINT('Ctrl Pts',(-1.13527256282102,24.0031999223435,3.31124536858058));
#4504=CARTESIAN_POINT('Ctrl Pts',(-2.21116140213284,24.1281999223435,2.94237295232722));
#4505=CARTESIAN_POINT('Ctrl Pts',(-2.86475599094322,24.2531999223435,2.01155730596855));
#4506=CARTESIAN_POINT('Ctrl Pts',(-3.51835057975361,24.3781999223435,1.08074165960988));
#4507=CARTESIAN_POINT('Ctrl Pts',(-3.5,24.5031999223435,-0.0564772772052956));
#4508=CARTESIAN_POINT('Ctrl Pts',(-3.48164942024639,24.6281999223435,-1.19369621402047));
#4509=CARTESIAN_POINT('Ctrl Pts',(-2.79836296968141,24.7531999223435,-2.10293946007877));
#4510=CARTESIAN_POINT('Ctrl Pts',(-2.11507651911643,24.8781999223436,-3.01218270613706));
#4511=CARTESIAN_POINT('Ctrl Pts',(-1.02784639780361,25.0031999223435,-3.3461502454855));
#4512=CARTESIAN_POINT('Ctrl Pts',(0.0593837235092011,25.1281999223435,-3.68011778483394));
#4513=CARTESIAN_POINT('Ctrl Pts',(1.13527256282102,25.2531999223435,-3.31124536858058));
#4514=CARTESIAN_POINT('Ctrl Pts',(2.21116140213284,25.3781999223435,-2.94237295232722));
#4515=CARTESIAN_POINT('Ctrl Pts',(2.86475599094322,25.5031999223436,-2.01155730596855));
#4516=CARTESIAN_POINT('Ctrl Pts',(3.51835057975361,25.6281999223435,-1.08074165960988));
#4517=CARTESIAN_POINT('Ctrl Pts',(3.5,25.7531999223436,0.0564772772052952));
#4518=CARTESIAN_POINT('Ctrl Pts',(3.48164942024639,25.8781999223435,1.19369621402047));
#4519=CARTESIAN_POINT('Ctrl Pts',(2.79836296968141,26.0031999223435,2.10293946007876));
#4520=CARTESIAN_POINT('Ctrl Pts',(2.11507651911643,26.1281999223436,3.01218270613706));
#4521=CARTESIAN_POINT('Ctrl Pts',(1.02784639780361,26.2531999223435,3.3461502454855));
#4522=CARTESIAN_POINT('Ctrl Pts',(-0.0593837235092006,26.3781999223435,
3.68011778483394));
#4523=CARTESIAN_POINT('Ctrl Pts',(-1.13527256282102,26.5031999223435,3.31124536858058));
#4524=CARTESIAN_POINT('Ctrl Pts',(-2.21116140213284,26.6281999223435,2.94237295232722));
#4525=CARTESIAN_POINT('Ctrl Pts',(-2.86475599094322,26.7531999223436,2.01155730596855));
#4526=CARTESIAN_POINT('Ctrl Pts',(-3.51835057975361,26.8781999223435,1.08074165960988));
#4527=CARTESIAN_POINT('Ctrl Pts',(-3.5,27.0031999223436,-0.0564772772052956));
#4528=CARTESIAN_POINT('Ctrl Pts',(-3.48164942024639,27.1281999223435,-1.19369621402047));
#4529=CARTESIAN_POINT('Ctrl Pts',(-2.79836296968141,27.2531999223435,-2.10293946007877));
#4530=CARTESIAN_POINT('Ctrl Pts',(-2.11507651911643,27.3781999223436,-3.01218270613706));
#4531=CARTESIAN_POINT('Ctrl Pts',(-1.02784639780361,27.5031999223435,-3.3461502454855));
#4532=CARTESIAN_POINT('Ctrl Pts',(0.0593837235092011,27.6281999223435,-3.68011778483394));
#4533=CARTESIAN_POINT('Ctrl Pts',(1.13527256282102,27.7531999223435,-3.31124536858058));
#4534=CARTESIAN_POINT('Ctrl Pts',(2.21116140213284,27.8781999223435,-2.94237295232722));
#4535=CARTESIAN_POINT('Ctrl Pts',(2.86475599094322,28.0031999223435,-2.01155730596855));
#4536=CARTESIAN_POINT('Ctrl Pts',(3.51835057975361,28.1281999223435,-1.08074165960988));
#4537=CARTESIAN_POINT('Ctrl Pts',(3.5,28.2531999223435,0.0564772772052952));
#4538=CARTESIAN_POINT('Ctrl Pts',(3.48164942024639,28.3781999223435,1.19369621402047));
#4539=CARTESIAN_POINT('Ctrl Pts',(2.79836296968141,28.5031999223435,2.10293946007876));
#4540=CARTESIAN_POINT('Ctrl Pts',(2.11507651911643,28.6281999223435,3.01218270613706));
#4541=CARTESIAN_POINT('Ctrl Pts',(1.02784639780361,28.7531999223435,3.3461502454855));
#4542=CARTESIAN_POINT('Ctrl Pts',(-0.0593837235092006,28.8781999223435,
3.68011778483394));
#4543=CARTESIAN_POINT('Ctrl Pts',(-1.13527256282102,29.0031999223435,3.31124536858058));
#4544=CARTESIAN_POINT('Ctrl Pts',(-2.21116140213284,29.1281999223435,2.94237295232722));
#4545=CARTESIAN_POINT('Ctrl Pts',(-2.86475599094322,29.2531999223435,2.01155730596855));
#4546=CARTESIAN_POINT('Ctrl Pts',(-3.51835057975361,29.3781999223435,1.08074165960988));
#4547=CARTESIAN_POINT('Ctrl Pts',(-3.5,29.5031999223435,-0.0564772772052956));
#4548=CARTESIAN_POINT('Ctrl Pts',(-3.48164942024639,29.6281999223435,-1.19369621402047));
#4549=CARTESIAN_POINT('Ctrl Pts',(-2.79836296968141,29.7531999223435,-2.10293946007877));
#4550=CARTESIAN_POINT('Ctrl Pts',(-2.11507651911643,29.8781999223435,-3.01218270613706));
#4551=CARTESIAN_POINT('Ctrl Pts',(-1.02784639780361,30.0031999223435,-3.3461502454855));
#4552=CARTESIAN_POINT('Ctrl Pts',(0.0593837235092011,30.1281999223435,-3.68011778483394));
#4553=CARTESIAN_POINT('Ctrl Pts',(1.13527256282102,30.2531999223435,-3.31124536858058));
#4554=CARTESIAN_POINT('Ctrl Pts',(2.21116140213284,30.3781999223435,-2.94237295232722));
#4555=CARTESIAN_POINT('Ctrl Pts',(2.86475599094322,30.5031999223435,-2.01155730596855));
#4556=CARTESIAN_POINT('Ctrl Pts',(3.51835057975361,30.6281999223435,-1.08074165960988));
#4557=CARTESIAN_POINT('Ctrl Pts',(3.5,30.7531999223435,0.0564772772052952));
#4558=CARTESIAN_POINT('Ctrl Pts',(3.48164942024639,30.8781999223435,1.19369621402047));
#4559=CARTESIAN_POINT('Ctrl Pts',(2.79836296968141,31.0031999223435,2.10293946007876));
#4560=CARTESIAN_POINT('Ctrl Pts',(2.11507651911643,31.1281999223435,3.01218270613706));
#4561=CARTESIAN_POINT('Ctrl Pts',(1.02784639780361,31.2531999223435,3.3461502454855));
#4562=CARTESIAN_POINT('Ctrl Pts',(-0.0593837235092006,31.3781999223435,
3.68011778483394));
#4563=CARTESIAN_POINT('Ctrl Pts',(-1.13527256282102,31.5031999223435,3.31124536858058));
#4564=CARTESIAN_POINT('Ctrl Pts',(-2.21116140213284,31.6281999223435,2.94237295232722));
#4565=CARTESIAN_POINT('Ctrl Pts',(-2.86475599094322,31.7531999223435,2.01155730596855));
#4566=CARTESIAN_POINT('Ctrl Pts',(-3.51835057975361,31.8781999223435,1.08074165960988));
#4567=CARTESIAN_POINT('Ctrl Pts',(-3.5,32.0031999223435,-0.0564772772052956));
#4568=CARTESIAN_POINT('Ctrl Pts',(-3.48164942024639,32.1281999223435,-1.19369621402047));
#4569=CARTESIAN_POINT('Ctrl Pts',(-2.79836296968141,32.2531999223435,-2.10293946007877));
#4570=CARTESIAN_POINT('Ctrl Pts',(-2.11507651911643,32.3781999223436,-3.01218270613706));
#4571=CARTESIAN_POINT('Ctrl Pts',(-1.02784639780361,32.5031999223435,-3.3461502454855));
#4572=CARTESIAN_POINT('Ctrl Pts',(0.0593837235092011,32.6281999223435,-3.68011778483394));
#4573=CARTESIAN_POINT('Ctrl Pts',(1.13527256282102,32.7531999223435,-3.31124536858058));
#4574=CARTESIAN_POINT('Ctrl Pts',(2.21116140213284,32.8781999223435,-2.94237295232722));
#4575=CARTESIAN_POINT('Ctrl Pts',(2.86475599094322,33.0031999223436,-2.01155730596855));
#4576=CARTESIAN_POINT('Ctrl Pts',(3.51835057975361,33.1281999223435,-1.08074165960988));
#4577=CARTESIAN_POINT('Ctrl Pts',(3.5,33.2531999223435,0.0564772772052952));
#4578=CARTESIAN_POINT('Ctrl Pts',(3.48164942024639,33.3781999223435,1.19369621402047));
#4579=CARTESIAN_POINT('Ctrl Pts',(2.79836296968141,33.5031999223435,2.10293946007876));
#4580=CARTESIAN_POINT('Ctrl Pts',(2.11507651911643,33.6281999223435,3.01218270613706));
#4581=CARTESIAN_POINT('Ctrl Pts',(1.02784639780361,33.7531999223435,3.3461502454855));
#4582=CARTESIAN_POINT('Ctrl Pts',(-0.0593837235092006,33.8781999223435,
3.68011778483394));
#4583=CARTESIAN_POINT('Ctrl Pts',(-1.13527256282102,34.0031999223435,3.31124536858058));
#4584=CARTESIAN_POINT('Ctrl Pts',(-2.21116140213284,34.1281999223436,2.94237295232722));
#4585=CARTESIAN_POINT('Ctrl Pts',(-2.86475599094322,34.2531999223436,2.01155730596855));
#4586=CARTESIAN_POINT('Ctrl Pts',(-3.51835057975361,34.3781999223435,1.08074165960988));
#4587=CARTESIAN_POINT('Ctrl Pts',(-3.5,34.5031999223435,-0.0564772772052956));
#4588=CARTESIAN_POINT('Ctrl Pts',(-3.48164942024639,34.6281999223435,-1.19369621402047));
#4589=CARTESIAN_POINT('Ctrl Pts',(-2.79836296968141,34.7531999223435,-2.10293946007877));
#4590=CARTESIAN_POINT('Ctrl Pts',(-2.11507651911643,34.8781999223436,-3.01218270613706));
#4591=CARTESIAN_POINT('Ctrl Pts',(-1.02784639780361,35.0031999223435,-3.3461502454855));
#4592=CARTESIAN_POINT('Ctrl Pts',(0.0593837235092011,35.1281999223435,-3.68011778483394));
#4593=CARTESIAN_POINT('Ctrl Pts',(1.13527256282102,35.2531999223435,-3.31124536858058));
#4594=CARTESIAN_POINT('Ctrl Pts',(2.21116140213284,35.3781999223435,-2.94237295232722));
#4595=CARTESIAN_POINT('Ctrl Pts',(2.86475599094322,35.5031999223436,-2.01155730596855));
#4596=CARTESIAN_POINT('Ctrl Pts',(3.51835057975361,35.6281999223435,-1.08074165960988));
#4597=CARTESIAN_POINT('Ctrl Pts',(3.5,35.7531999223435,0.0564772772052952));
#4598=CARTESIAN_POINT('Ctrl Pts',(3.48164942024639,35.8781999223435,1.19369621402047));
#4599=CARTESIAN_POINT('Ctrl Pts',(2.79836296968141,36.0031999223435,2.10293946007876));
#4600=CARTESIAN_POINT('Ctrl Pts',(2.11507651911643,36.1281999223436,3.01218270613706));
#4601=CARTESIAN_POINT('Ctrl Pts',(1.02784639780361,36.2531999223435,3.3461502454855));
#4602=CARTESIAN_POINT('Ctrl Pts',(-0.0593837235092006,36.3781999223436,
3.68011778483394));
#4603=CARTESIAN_POINT('Ctrl Pts',(-1.13527256282102,36.5031999223435,3.31124536858058));
#4604=CARTESIAN_POINT('Ctrl Pts',(-2.21116140213284,36.6281999223435,2.94237295232722));
#4605=CARTESIAN_POINT('Ctrl Pts',(-2.86475599094322,36.7531999223435,2.01155730596855));
#4606=CARTESIAN_POINT('Ctrl Pts',(-3.51835057975361,36.8781999223435,1.08074165960988));
#4607=CARTESIAN_POINT('Ctrl Pts',(-3.5,37.0031999223435,-0.0564772772052956));
#4608=CARTESIAN_POINT('Ctrl Pts',(-3.48164942024639,37.1281999223435,-1.19369621402047));
#4609=CARTESIAN_POINT('Ctrl Pts',(-2.79836296968141,37.2531999223435,-2.10293946007877));
#4610=CARTESIAN_POINT('Ctrl Pts',(-2.11507651911643,37.3781999223435,-3.01218270613706));
#4611=CARTESIAN_POINT('Ctrl Pts',(-1.02784639780361,37.5031999223435,-3.3461502454855));
#4612=CARTESIAN_POINT('Ctrl Pts',(0.0593837235092011,37.6281999223435,-3.68011778483394));
#4613=CARTESIAN_POINT('Ctrl Pts',(1.13527256282102,37.7531999223435,-3.31124536858058));
#4614=CARTESIAN_POINT('Ctrl Pts',(2.21116140213284,37.8781999223435,-2.94237295232722));
#4615=CARTESIAN_POINT('Ctrl Pts',(2.86475599094322,38.0031999223435,-2.01155730596855));
#4616=CARTESIAN_POINT('Ctrl Pts',(3.51835057975361,38.1281999223435,-1.08074165960988));
#4617=CARTESIAN_POINT('Ctrl Pts',(3.5,38.2531999223435,0.0564772772052952));
#4618=CARTESIAN_POINT('Ctrl Pts',(3.48164942024639,38.3781999223435,1.19369621402047));
#4619=CARTESIAN_POINT('Ctrl Pts',(2.79836296968141,38.5031999223435,2.10293946007876));
#4620=CARTESIAN_POINT('Ctrl Pts',(2.11507651911643,38.6281999223436,3.01218270613706));
#4621=CARTESIAN_POINT('Ctrl Pts',(1.02784639780361,38.7531999223435,3.3461502454855));
#4622=CARTESIAN_POINT('Ctrl Pts',(-0.0593837235092006,38.8781999223435,
3.68011778483394));
#4623=CARTESIAN_POINT('Ctrl Pts',(-1.13527256282102,39.0031999223435,3.31124536858058));
#4624=CARTESIAN_POINT('Ctrl Pts',(-2.21116140213284,39.1281999223435,2.94237295232722));
#4625=CARTESIAN_POINT('Ctrl Pts',(-2.86475599094322,39.2531999223436,2.01155730596855));
#4626=CARTESIAN_POINT('Ctrl Pts',(-3.51835057975361,39.3781999223435,1.08074165960988));
#4627=CARTESIAN_POINT('Ctrl Pts',(-3.5,39.5031999223435,-0.0564772772052956));
#4628=CARTESIAN_POINT('Ctrl Pts',(-4.5,14.5031999223435,-0.0564772772052853));
#4629=CARTESIAN_POINT('Ctrl Pts',(-4.4816494202464,14.6281999223435,-1.51861591025336));
#4630=CARTESIAN_POINT('Ctrl Pts',(-3.60737996405636,14.7531999223435,-2.69072471237123));
#4631=CARTESIAN_POINT('Ctrl Pts',(-2.73311050786633,14.8781999223435,-3.8628335144891));
#4632=CARTESIAN_POINT('Ctrl Pts',(-1.33686339217857,15.0031999223435,-4.29720676178065));
#4633=CARTESIAN_POINT('Ctrl Pts',(0.0593837235091902,15.1281999223435,-4.7315800090722));
#4634=CARTESIAN_POINT('Ctrl Pts',(1.44428955719596,15.2531999223435,-4.26230188487573));
#4635=CARTESIAN_POINT('Ctrl Pts',(2.82919539088272,15.3781999223435,-3.79302376067926));
#4636=CARTESIAN_POINT('Ctrl Pts',(3.67377298531816,15.5031999223435,-2.59934255826103));
#4637=CARTESIAN_POINT('Ctrl Pts',(4.5183505797536,15.6281999223435,-1.40566135584279));
#4638=CARTESIAN_POINT('Ctrl Pts',(4.5,15.7531999223435,0.0564772772052848));
#4639=CARTESIAN_POINT('Ctrl Pts',(4.4816494202464,15.8781999223435,1.51861591025336));
#4640=CARTESIAN_POINT('Ctrl Pts',(3.60737996405636,16.0031999223435,2.69072471237123));
#4641=CARTESIAN_POINT('Ctrl Pts',(2.73311050786633,16.1281999223435,3.8628335144891));
#4642=CARTESIAN_POINT('Ctrl Pts',(1.33686339217857,16.2531999223435,4.29720676178065));
#4643=CARTESIAN_POINT('Ctrl Pts',(-0.0593837235091896,16.3781999223435,
4.7315800090722));
#4644=CARTESIAN_POINT('Ctrl Pts',(-1.44428955719596,16.5031999223435,4.26230188487573));
#4645=CARTESIAN_POINT('Ctrl Pts',(-2.82919539088272,16.6281999223435,3.79302376067927));
#4646=CARTESIAN_POINT('Ctrl Pts',(-3.67377298531816,16.7531999223435,2.59934255826103));
#4647=CARTESIAN_POINT('Ctrl Pts',(-4.5183505797536,16.8781999223435,1.40566135584279));
#4648=CARTESIAN_POINT('Ctrl Pts',(-4.5,17.0031999223435,-0.0564772772052853));
#4649=CARTESIAN_POINT('Ctrl Pts',(-4.4816494202464,17.1281999223435,-1.51861591025336));
#4650=CARTESIAN_POINT('Ctrl Pts',(-3.60737996405636,17.2531999223435,-2.69072471237123));
#4651=CARTESIAN_POINT('Ctrl Pts',(-2.73311050786633,17.3781999223435,-3.8628335144891));
#4652=CARTESIAN_POINT('Ctrl Pts',(-1.33686339217857,17.5031999223435,-4.29720676178065));
#4653=CARTESIAN_POINT('Ctrl Pts',(0.0593837235091902,17.6281999223435,-4.7315800090722));
#4654=CARTESIAN_POINT('Ctrl Pts',(1.44428955719596,17.7531999223435,-4.26230188487573));
#4655=CARTESIAN_POINT('Ctrl Pts',(2.82919539088272,17.8781999223435,-3.79302376067926));
#4656=CARTESIAN_POINT('Ctrl Pts',(3.67377298531816,18.0031999223435,-2.59934255826103));
#4657=CARTESIAN_POINT('Ctrl Pts',(4.5183505797536,18.1281999223435,-1.40566135584279));
#4658=CARTESIAN_POINT('Ctrl Pts',(4.5,18.2531999223435,0.0564772772052848));
#4659=CARTESIAN_POINT('Ctrl Pts',(4.4816494202464,18.3781999223435,1.51861591025336));
#4660=CARTESIAN_POINT('Ctrl Pts',(3.60737996405636,18.5031999223435,2.69072471237123));
#4661=CARTESIAN_POINT('Ctrl Pts',(2.73311050786633,18.6281999223435,3.8628335144891));
#4662=CARTESIAN_POINT('Ctrl Pts',(1.33686339217857,18.7531999223435,4.29720676178065));
#4663=CARTESIAN_POINT('Ctrl Pts',(-0.0593837235091896,18.8781999223435,
4.7315800090722));
#4664=CARTESIAN_POINT('Ctrl Pts',(-1.44428955719596,19.0031999223435,4.26230188487573));
#4665=CARTESIAN_POINT('Ctrl Pts',(-2.82919539088272,19.1281999223435,3.79302376067927));
#4666=CARTESIAN_POINT('Ctrl Pts',(-3.67377298531816,19.2531999223435,2.59934255826103));
#4667=CARTESIAN_POINT('Ctrl Pts',(-4.5183505797536,19.3781999223435,1.40566135584279));
#4668=CARTESIAN_POINT('Ctrl Pts',(-4.5,19.5031999223435,-0.0564772772052853));
#4669=CARTESIAN_POINT('Ctrl Pts',(-4.4816494202464,19.6281999223435,-1.51861591025336));
#4670=CARTESIAN_POINT('Ctrl Pts',(-3.60737996405636,19.7531999223435,-2.69072471237123));
#4671=CARTESIAN_POINT('Ctrl Pts',(-2.73311050786633,19.8781999223435,-3.8628335144891));
#4672=CARTESIAN_POINT('Ctrl Pts',(-1.33686339217857,20.0031999223435,-4.29720676178065));
#4673=CARTESIAN_POINT('Ctrl Pts',(0.0593837235091902,20.1281999223435,-4.7315800090722));
#4674=CARTESIAN_POINT('Ctrl Pts',(1.44428955719596,20.2531999223435,-4.26230188487573));
#4675=CARTESIAN_POINT('Ctrl Pts',(2.82919539088272,20.3781999223435,-3.79302376067926));
#4676=CARTESIAN_POINT('Ctrl Pts',(3.67377298531816,20.5031999223435,-2.59934255826103));
#4677=CARTESIAN_POINT('Ctrl Pts',(4.5183505797536,20.6281999223435,-1.40566135584279));
#4678=CARTESIAN_POINT('Ctrl Pts',(4.5,20.7531999223435,0.0564772772052848));
#4679=CARTESIAN_POINT('Ctrl Pts',(4.4816494202464,20.8781999223435,1.51861591025336));
#4680=CARTESIAN_POINT('Ctrl Pts',(3.60737996405636,21.0031999223435,2.69072471237123));
#4681=CARTESIAN_POINT('Ctrl Pts',(2.73311050786633,21.1281999223435,3.8628335144891));
#4682=CARTESIAN_POINT('Ctrl Pts',(1.33686339217857,21.2531999223435,4.29720676178065));
#4683=CARTESIAN_POINT('Ctrl Pts',(-0.0593837235091896,21.3781999223435,
4.7315800090722));
#4684=CARTESIAN_POINT('Ctrl Pts',(-1.44428955719596,21.5031999223435,4.26230188487573));
#4685=CARTESIAN_POINT('Ctrl Pts',(-2.82919539088272,21.6281999223435,3.79302376067927));
#4686=CARTESIAN_POINT('Ctrl Pts',(-3.67377298531816,21.7531999223435,2.59934255826103));
#4687=CARTESIAN_POINT('Ctrl Pts',(-4.5183505797536,21.8781999223435,1.40566135584279));
#4688=CARTESIAN_POINT('Ctrl Pts',(-4.5,22.0031999223435,-0.0564772772052853));
#4689=CARTESIAN_POINT('Ctrl Pts',(-4.4816494202464,22.1281999223435,-1.51861591025336));
#4690=CARTESIAN_POINT('Ctrl Pts',(-3.60737996405636,22.2531999223435,-2.69072471237123));
#4691=CARTESIAN_POINT('Ctrl Pts',(-2.73311050786633,22.3781999223435,-3.8628335144891));
#4692=CARTESIAN_POINT('Ctrl Pts',(-1.33686339217857,22.5031999223435,-4.29720676178065));
#4693=CARTESIAN_POINT('Ctrl Pts',(0.0593837235091902,22.6281999223435,-4.7315800090722));
#4694=CARTESIAN_POINT('Ctrl Pts',(1.44428955719596,22.7531999223435,-4.26230188487573));
#4695=CARTESIAN_POINT('Ctrl Pts',(2.82919539088272,22.8781999223435,-3.79302376067926));
#4696=CARTESIAN_POINT('Ctrl Pts',(3.67377298531816,23.0031999223435,-2.59934255826103));
#4697=CARTESIAN_POINT('Ctrl Pts',(4.5183505797536,23.1281999223435,-1.40566135584279));
#4698=CARTESIAN_POINT('Ctrl Pts',(4.5,23.2531999223435,0.0564772772052848));
#4699=CARTESIAN_POINT('Ctrl Pts',(4.4816494202464,23.3781999223435,1.51861591025336));
#4700=CARTESIAN_POINT('Ctrl Pts',(3.60737996405636,23.5031999223435,2.69072471237123));
#4701=CARTESIAN_POINT('Ctrl Pts',(2.73311050786633,23.6281999223435,3.8628335144891));
#4702=CARTESIAN_POINT('Ctrl Pts',(1.33686339217857,23.7531999223435,4.29720676178065));
#4703=CARTESIAN_POINT('Ctrl Pts',(-0.0593837235091896,23.8781999223435,
4.7315800090722));
#4704=CARTESIAN_POINT('Ctrl Pts',(-1.44428955719596,24.0031999223435,4.26230188487573));
#4705=CARTESIAN_POINT('Ctrl Pts',(-2.82919539088272,24.1281999223435,3.79302376067927));
#4706=CARTESIAN_POINT('Ctrl Pts',(-3.67377298531816,24.2531999223435,2.59934255826103));
#4707=CARTESIAN_POINT('Ctrl Pts',(-4.5183505797536,24.3781999223435,1.40566135584279));
#4708=CARTESIAN_POINT('Ctrl Pts',(-4.5,24.5031999223436,-0.0564772772052853));
#4709=CARTESIAN_POINT('Ctrl Pts',(-4.4816494202464,24.6281999223435,-1.51861591025336));
#4710=CARTESIAN_POINT('Ctrl Pts',(-3.60737996405636,24.7531999223435,-2.69072471237123));
#4711=CARTESIAN_POINT('Ctrl Pts',(-2.73311050786633,24.8781999223436,-3.8628335144891));
#4712=CARTESIAN_POINT('Ctrl Pts',(-1.33686339217857,25.0031999223435,-4.29720676178065));
#4713=CARTESIAN_POINT('Ctrl Pts',(0.0593837235091902,25.1281999223435,-4.7315800090722));
#4714=CARTESIAN_POINT('Ctrl Pts',(1.44428955719596,25.2531999223435,-4.26230188487573));
#4715=CARTESIAN_POINT('Ctrl Pts',(2.82919539088272,25.3781999223435,-3.79302376067926));
#4716=CARTESIAN_POINT('Ctrl Pts',(3.67377298531816,25.5031999223435,-2.59934255826103));
#4717=CARTESIAN_POINT('Ctrl Pts',(4.5183505797536,25.6281999223435,-1.40566135584279));
#4718=CARTESIAN_POINT('Ctrl Pts',(4.5,25.7531999223436,0.0564772772052848));
#4719=CARTESIAN_POINT('Ctrl Pts',(4.4816494202464,25.8781999223436,1.51861591025336));
#4720=CARTESIAN_POINT('Ctrl Pts',(3.60737996405636,26.0031999223435,2.69072471237123));
#4721=CARTESIAN_POINT('Ctrl Pts',(2.73311050786633,26.1281999223435,3.8628335144891));
#4722=CARTESIAN_POINT('Ctrl Pts',(1.33686339217857,26.2531999223435,4.29720676178065));
#4723=CARTESIAN_POINT('Ctrl Pts',(-0.0593837235091896,26.3781999223436,
4.7315800090722));
#4724=CARTESIAN_POINT('Ctrl Pts',(-1.44428955719596,26.5031999223435,4.26230188487573));
#4725=CARTESIAN_POINT('Ctrl Pts',(-2.82919539088272,26.6281999223435,3.79302376067927));
#4726=CARTESIAN_POINT('Ctrl Pts',(-3.67377298531816,26.7531999223436,2.59934255826103));
#4727=CARTESIAN_POINT('Ctrl Pts',(-4.5183505797536,26.8781999223435,1.40566135584279));
#4728=CARTESIAN_POINT('Ctrl Pts',(-4.5,27.0031999223436,-0.0564772772052853));
#4729=CARTESIAN_POINT('Ctrl Pts',(-4.4816494202464,27.1281999223436,-1.51861591025336));
#4730=CARTESIAN_POINT('Ctrl Pts',(-3.60737996405636,27.2531999223435,-2.69072471237123));
#4731=CARTESIAN_POINT('Ctrl Pts',(-2.73311050786633,27.3781999223436,-3.8628335144891));
#4732=CARTESIAN_POINT('Ctrl Pts',(-1.33686339217857,27.5031999223435,-4.29720676178065));
#4733=CARTESIAN_POINT('Ctrl Pts',(0.0593837235091902,27.6281999223435,-4.7315800090722));
#4734=CARTESIAN_POINT('Ctrl Pts',(1.44428955719596,27.7531999223435,-4.26230188487573));
#4735=CARTESIAN_POINT('Ctrl Pts',(2.82919539088272,27.8781999223435,-3.79302376067926));
#4736=CARTESIAN_POINT('Ctrl Pts',(3.67377298531816,28.0031999223436,-2.59934255826103));
#4737=CARTESIAN_POINT('Ctrl Pts',(4.5183505797536,28.1281999223435,-1.40566135584279));
#4738=CARTESIAN_POINT('Ctrl Pts',(4.5,28.2531999223435,0.0564772772052848));
#4739=CARTESIAN_POINT('Ctrl Pts',(4.4816494202464,28.3781999223436,1.51861591025336));
#4740=CARTESIAN_POINT('Ctrl Pts',(3.60737996405636,28.5031999223435,2.69072471237123));
#4741=CARTESIAN_POINT('Ctrl Pts',(2.73311050786633,28.6281999223435,3.8628335144891));
#4742=CARTESIAN_POINT('Ctrl Pts',(1.33686339217857,28.7531999223435,4.29720676178065));
#4743=CARTESIAN_POINT('Ctrl Pts',(-0.0593837235091896,28.8781999223435,
4.7315800090722));
#4744=CARTESIAN_POINT('Ctrl Pts',(-1.44428955719596,29.0031999223435,4.26230188487573));
#4745=CARTESIAN_POINT('Ctrl Pts',(-2.82919539088272,29.1281999223435,3.79302376067927));
#4746=CARTESIAN_POINT('Ctrl Pts',(-3.67377298531816,29.2531999223435,2.59934255826103));
#4747=CARTESIAN_POINT('Ctrl Pts',(-4.5183505797536,29.3781999223436,1.40566135584279));
#4748=CARTESIAN_POINT('Ctrl Pts',(-4.5,29.5031999223435,-0.0564772772052853));
#4749=CARTESIAN_POINT('Ctrl Pts',(-4.4816494202464,29.6281999223435,-1.51861591025336));
#4750=CARTESIAN_POINT('Ctrl Pts',(-3.60737996405636,29.7531999223435,-2.69072471237123));
#4751=CARTESIAN_POINT('Ctrl Pts',(-2.73311050786633,29.8781999223435,-3.8628335144891));
#4752=CARTESIAN_POINT('Ctrl Pts',(-1.33686339217857,30.0031999223435,-4.29720676178065));
#4753=CARTESIAN_POINT('Ctrl Pts',(0.0593837235091902,30.1281999223435,-4.7315800090722));
#4754=CARTESIAN_POINT('Ctrl Pts',(1.44428955719596,30.2531999223435,-4.26230188487573));
#4755=CARTESIAN_POINT('Ctrl Pts',(2.82919539088272,30.3781999223435,-3.79302376067926));
#4756=CARTESIAN_POINT('Ctrl Pts',(3.67377298531816,30.5031999223435,-2.59934255826103));
#4757=CARTESIAN_POINT('Ctrl Pts',(4.5183505797536,30.6281999223435,-1.40566135584279));
#4758=CARTESIAN_POINT('Ctrl Pts',(4.5,30.7531999223435,0.0564772772052848));
#4759=CARTESIAN_POINT('Ctrl Pts',(4.4816494202464,30.8781999223435,1.51861591025336));
#4760=CARTESIAN_POINT('Ctrl Pts',(3.60737996405636,31.0031999223435,2.69072471237123));
#4761=CARTESIAN_POINT('Ctrl Pts',(2.73311050786633,31.1281999223435,3.8628335144891));
#4762=CARTESIAN_POINT('Ctrl Pts',(1.33686339217857,31.2531999223435,4.29720676178065));
#4763=CARTESIAN_POINT('Ctrl Pts',(-0.0593837235091896,31.3781999223435,
4.7315800090722));
#4764=CARTESIAN_POINT('Ctrl Pts',(-1.44428955719596,31.5031999223435,4.26230188487573));
#4765=CARTESIAN_POINT('Ctrl Pts',(-2.82919539088272,31.6281999223435,3.79302376067927));
#4766=CARTESIAN_POINT('Ctrl Pts',(-3.67377298531816,31.7531999223436,2.59934255826103));
#4767=CARTESIAN_POINT('Ctrl Pts',(-4.5183505797536,31.8781999223435,1.40566135584279));
#4768=CARTESIAN_POINT('Ctrl Pts',(-4.5,32.0031999223435,-0.0564772772052853));
#4769=CARTESIAN_POINT('Ctrl Pts',(-4.4816494202464,32.1281999223435,-1.51861591025336));
#4770=CARTESIAN_POINT('Ctrl Pts',(-3.60737996405636,32.2531999223435,-2.69072471237123));
#4771=CARTESIAN_POINT('Ctrl Pts',(-2.73311050786633,32.3781999223435,-3.8628335144891));
#4772=CARTESIAN_POINT('Ctrl Pts',(-1.33686339217857,32.5031999223435,-4.29720676178065));
#4773=CARTESIAN_POINT('Ctrl Pts',(0.0593837235091902,32.6281999223435,-4.7315800090722));
#4774=CARTESIAN_POINT('Ctrl Pts',(1.44428955719596,32.7531999223435,-4.26230188487573));
#4775=CARTESIAN_POINT('Ctrl Pts',(2.82919539088272,32.8781999223435,-3.79302376067926));
#4776=CARTESIAN_POINT('Ctrl Pts',(3.67377298531816,33.0031999223436,-2.59934255826103));
#4777=CARTESIAN_POINT('Ctrl Pts',(4.5183505797536,33.1281999223435,-1.40566135584279));
#4778=CARTESIAN_POINT('Ctrl Pts',(4.5,33.2531999223435,0.0564772772052848));
#4779=CARTESIAN_POINT('Ctrl Pts',(4.4816494202464,33.3781999223435,1.51861591025336));
#4780=CARTESIAN_POINT('Ctrl Pts',(3.60737996405636,33.5031999223435,2.69072471237123));
#4781=CARTESIAN_POINT('Ctrl Pts',(2.73311050786633,33.6281999223436,3.8628335144891));
#4782=CARTESIAN_POINT('Ctrl Pts',(1.33686339217857,33.7531999223435,4.29720676178065));
#4783=CARTESIAN_POINT('Ctrl Pts',(-0.0593837235091896,33.8781999223435,
4.7315800090722));
#4784=CARTESIAN_POINT('Ctrl Pts',(-1.44428955719596,34.0031999223435,4.26230188487573));
#4785=CARTESIAN_POINT('Ctrl Pts',(-2.82919539088272,34.1281999223435,3.79302376067927));
#4786=CARTESIAN_POINT('Ctrl Pts',(-3.67377298531816,34.2531999223435,2.59934255826103));
#4787=CARTESIAN_POINT('Ctrl Pts',(-4.5183505797536,34.3781999223435,1.40566135584279));
#4788=CARTESIAN_POINT('Ctrl Pts',(-4.5,34.5031999223435,-0.0564772772052853));
#4789=CARTESIAN_POINT('Ctrl Pts',(-4.4816494202464,34.6281999223435,-1.51861591025336));
#4790=CARTESIAN_POINT('Ctrl Pts',(-3.60737996405636,34.7531999223435,-2.69072471237123));
#4791=CARTESIAN_POINT('Ctrl Pts',(-2.73311050786633,34.8781999223436,-3.8628335144891));
#4792=CARTESIAN_POINT('Ctrl Pts',(-1.33686339217857,35.0031999223435,-4.29720676178065));
#4793=CARTESIAN_POINT('Ctrl Pts',(0.0593837235091902,35.1281999223435,-4.7315800090722));
#4794=CARTESIAN_POINT('Ctrl Pts',(1.44428955719596,35.2531999223435,-4.26230188487573));
#4795=CARTESIAN_POINT('Ctrl Pts',(2.82919539088272,35.3781999223435,-3.79302376067926));
#4796=CARTESIAN_POINT('Ctrl Pts',(3.67377298531816,35.5031999223436,-2.59934255826103));
#4797=CARTESIAN_POINT('Ctrl Pts',(4.5183505797536,35.6281999223435,-1.40566135584279));
#4798=CARTESIAN_POINT('Ctrl Pts',(4.5,35.7531999223435,0.0564772772052848));
#4799=CARTESIAN_POINT('Ctrl Pts',(4.4816494202464,35.8781999223435,1.51861591025336));
#4800=CARTESIAN_POINT('Ctrl Pts',(3.60737996405636,36.0031999223435,2.69072471237123));
#4801=CARTESIAN_POINT('Ctrl Pts',(2.73311050786633,36.1281999223436,3.8628335144891));
#4802=CARTESIAN_POINT('Ctrl Pts',(1.33686339217857,36.2531999223435,4.29720676178065));
#4803=CARTESIAN_POINT('Ctrl Pts',(-0.0593837235091896,36.3781999223435,
4.7315800090722));
#4804=CARTESIAN_POINT('Ctrl Pts',(-1.44428955719596,36.5031999223435,4.26230188487573));
#4805=CARTESIAN_POINT('Ctrl Pts',(-2.82919539088272,36.6281999223435,3.79302376067927));
#4806=CARTESIAN_POINT('Ctrl Pts',(-3.67377298531816,36.7531999223435,2.59934255826103));
#4807=CARTESIAN_POINT('Ctrl Pts',(-4.5183505797536,36.8781999223435,1.40566135584279));
#4808=CARTESIAN_POINT('Ctrl Pts',(-4.5,37.0031999223435,-0.0564772772052853));
#4809=CARTESIAN_POINT('Ctrl Pts',(-4.4816494202464,37.1281999223435,-1.51861591025336));
#4810=CARTESIAN_POINT('Ctrl Pts',(-3.60737996405636,37.2531999223435,-2.69072471237123));
#4811=CARTESIAN_POINT('Ctrl Pts',(-2.73311050786633,37.3781999223436,-3.8628335144891));
#4812=CARTESIAN_POINT('Ctrl Pts',(-1.33686339217857,37.5031999223435,-4.29720676178065));
#4813=CARTESIAN_POINT('Ctrl Pts',(0.0593837235091902,37.6281999223435,-4.7315800090722));
#4814=CARTESIAN_POINT('Ctrl Pts',(1.44428955719596,37.7531999223435,-4.26230188487573));
#4815=CARTESIAN_POINT('Ctrl Pts',(2.82919539088272,37.8781999223435,-3.79302376067926));
#4816=CARTESIAN_POINT('Ctrl Pts',(3.67377298531816,38.0031999223435,-2.59934255826103));
#4817=CARTESIAN_POINT('Ctrl Pts',(4.5183505797536,38.1281999223435,-1.40566135584279));
#4818=CARTESIAN_POINT('Ctrl Pts',(4.5,38.2531999223435,0.0564772772052848));
#4819=CARTESIAN_POINT('Ctrl Pts',(4.4816494202464,38.3781999223435,1.51861591025336));
#4820=CARTESIAN_POINT('Ctrl Pts',(3.60737996405636,38.5031999223435,2.69072471237123));
#4821=CARTESIAN_POINT('Ctrl Pts',(2.73311050786633,38.6281999223436,3.8628335144891));
#4822=CARTESIAN_POINT('Ctrl Pts',(1.33686339217857,38.7531999223435,4.29720676178065));
#4823=CARTESIAN_POINT('Ctrl Pts',(-0.0593837235091896,38.8781999223435,
4.7315800090722));
#4824=CARTESIAN_POINT('Ctrl Pts',(-1.44428955719596,39.0031999223435,4.26230188487573));
#4825=CARTESIAN_POINT('Ctrl Pts',(-2.82919539088272,39.1281999223435,3.79302376067927));
#4826=CARTESIAN_POINT('Ctrl Pts',(-3.67377298531816,39.2531999223436,2.59934255826103));
#4827=CARTESIAN_POINT('Ctrl Pts',(-4.5183505797536,39.3781999223435,1.40566135584279));
#4828=CARTESIAN_POINT('Ctrl Pts',(-4.5,39.5031999223435,-0.0564772772052853));
#4829=CARTESIAN_POINT('Ctrl Pts',(-4.5,15.4968000776565,0.0564772772053793));
#4830=CARTESIAN_POINT('Ctrl Pts',(-4.51835057975363,15.6218000776565,-1.4056613558427));
#4831=CARTESIAN_POINT('Ctrl Pts',(-3.67377298531822,15.7468000776565,-2.59934255826095));
#4832=CARTESIAN_POINT('Ctrl Pts',(-2.82919539088281,15.8718000776565,-3.79302376067921));
#4833=CARTESIAN_POINT('Ctrl Pts',(-1.44428955719605,15.9968000776565,-4.2623018848757));
#4834=CARTESIAN_POINT('Ctrl Pts',(-0.0593837235092896,16.1218000776565,
-4.7315800090722));
#4835=CARTESIAN_POINT('Ctrl Pts',(1.33686339217848,16.2468000776565,-4.29720676178068));
#4836=CARTESIAN_POINT('Ctrl Pts',(2.73311050786625,16.3718000776565,-3.86283351448915));
#4837=CARTESIAN_POINT('Ctrl Pts',(3.60737996405631,16.4968000776565,-2.69072471237131));
#4838=CARTESIAN_POINT('Ctrl Pts',(4.48164942024637,16.6218000776565,-1.51861591025346));
#4839=CARTESIAN_POINT('Ctrl Pts',(4.5,16.7468000776565,-0.0564772772053798));
#4840=CARTESIAN_POINT('Ctrl Pts',(4.51835057975363,16.8718000776565,1.4056613558427));
#4841=CARTESIAN_POINT('Ctrl Pts',(3.67377298531822,16.9968000776565,2.59934255826095));
#4842=CARTESIAN_POINT('Ctrl Pts',(2.82919539088281,17.1218000776565,3.7930237606792));
#4843=CARTESIAN_POINT('Ctrl Pts',(1.44428955719605,17.2468000776565,4.2623018848757));
#4844=CARTESIAN_POINT('Ctrl Pts',(0.0593837235092902,17.3718000776565,4.7315800090722));
#4845=CARTESIAN_POINT('Ctrl Pts',(-1.33686339217848,17.4968000776565,4.29720676178068));
#4846=CARTESIAN_POINT('Ctrl Pts',(-2.73311050786625,17.6218000776565,3.86283351448915));
#4847=CARTESIAN_POINT('Ctrl Pts',(-3.60737996405631,17.7468000776565,2.69072471237131));
#4848=CARTESIAN_POINT('Ctrl Pts',(-4.48164942024637,17.8718000776565,1.51861591025346));
#4849=CARTESIAN_POINT('Ctrl Pts',(-4.5,17.9968000776565,0.0564772772053793));
#4850=CARTESIAN_POINT('Ctrl Pts',(-4.51835057975363,18.1218000776565,-1.4056613558427));
#4851=CARTESIAN_POINT('Ctrl Pts',(-3.67377298531822,18.2468000776565,-2.59934255826095));
#4852=CARTESIAN_POINT('Ctrl Pts',(-2.82919539088281,18.3718000776565,-3.79302376067921));
#4853=CARTESIAN_POINT('Ctrl Pts',(-1.44428955719605,18.4968000776565,-4.2623018848757));
#4854=CARTESIAN_POINT('Ctrl Pts',(-0.0593837235092896,18.6218000776565,
-4.7315800090722));
#4855=CARTESIAN_POINT('Ctrl Pts',(1.33686339217848,18.7468000776565,-4.29720676178068));
#4856=CARTESIAN_POINT('Ctrl Pts',(2.73311050786625,18.8718000776565,-3.86283351448915));
#4857=CARTESIAN_POINT('Ctrl Pts',(3.60737996405631,18.9968000776565,-2.69072471237131));
#4858=CARTESIAN_POINT('Ctrl Pts',(4.48164942024637,19.1218000776565,-1.51861591025346));
#4859=CARTESIAN_POINT('Ctrl Pts',(4.5,19.2468000776565,-0.0564772772053798));
#4860=CARTESIAN_POINT('Ctrl Pts',(4.51835057975363,19.3718000776565,1.4056613558427));
#4861=CARTESIAN_POINT('Ctrl Pts',(3.67377298531822,19.4968000776565,2.59934255826095));
#4862=CARTESIAN_POINT('Ctrl Pts',(2.82919539088281,19.6218000776565,3.7930237606792));
#4863=CARTESIAN_POINT('Ctrl Pts',(1.44428955719605,19.7468000776565,4.2623018848757));
#4864=CARTESIAN_POINT('Ctrl Pts',(0.0593837235092902,19.8718000776565,4.7315800090722));
#4865=CARTESIAN_POINT('Ctrl Pts',(-1.33686339217848,19.9968000776565,4.29720676178068));
#4866=CARTESIAN_POINT('Ctrl Pts',(-2.73311050786625,20.1218000776565,3.86283351448915));
#4867=CARTESIAN_POINT('Ctrl Pts',(-3.60737996405631,20.2468000776565,2.69072471237131));
#4868=CARTESIAN_POINT('Ctrl Pts',(-4.48164942024637,20.3718000776565,1.51861591025346));
#4869=CARTESIAN_POINT('Ctrl Pts',(-4.5,20.4968000776565,0.0564772772053793));
#4870=CARTESIAN_POINT('Ctrl Pts',(-4.51835057975363,20.6218000776565,-1.4056613558427));
#4871=CARTESIAN_POINT('Ctrl Pts',(-3.67377298531822,20.7468000776565,-2.59934255826095));
#4872=CARTESIAN_POINT('Ctrl Pts',(-2.82919539088281,20.8718000776565,-3.79302376067921));
#4873=CARTESIAN_POINT('Ctrl Pts',(-1.44428955719605,20.9968000776565,-4.2623018848757));
#4874=CARTESIAN_POINT('Ctrl Pts',(-0.0593837235092896,21.1218000776565,
-4.7315800090722));
#4875=CARTESIAN_POINT('Ctrl Pts',(1.33686339217848,21.2468000776565,-4.29720676178068));
#4876=CARTESIAN_POINT('Ctrl Pts',(2.73311050786625,21.3718000776565,-3.86283351448915));
#4877=CARTESIAN_POINT('Ctrl Pts',(3.60737996405631,21.4968000776565,-2.69072471237131));
#4878=CARTESIAN_POINT('Ctrl Pts',(4.48164942024637,21.6218000776565,-1.51861591025346));
#4879=CARTESIAN_POINT('Ctrl Pts',(4.5,21.7468000776565,-0.0564772772053798));
#4880=CARTESIAN_POINT('Ctrl Pts',(4.51835057975363,21.8718000776565,1.4056613558427));
#4881=CARTESIAN_POINT('Ctrl Pts',(3.67377298531822,21.9968000776565,2.59934255826095));
#4882=CARTESIAN_POINT('Ctrl Pts',(2.82919539088281,22.1218000776565,3.7930237606792));
#4883=CARTESIAN_POINT('Ctrl Pts',(1.44428955719605,22.2468000776565,4.2623018848757));
#4884=CARTESIAN_POINT('Ctrl Pts',(0.0593837235092902,22.3718000776565,4.7315800090722));
#4885=CARTESIAN_POINT('Ctrl Pts',(-1.33686339217848,22.4968000776565,4.29720676178068));
#4886=CARTESIAN_POINT('Ctrl Pts',(-2.73311050786625,22.6218000776565,3.86283351448915));
#4887=CARTESIAN_POINT('Ctrl Pts',(-3.60737996405631,22.7468000776565,2.69072471237131));
#4888=CARTESIAN_POINT('Ctrl Pts',(-4.48164942024637,22.8718000776565,1.51861591025346));
#4889=CARTESIAN_POINT('Ctrl Pts',(-4.5,22.9968000776565,0.0564772772053793));
#4890=CARTESIAN_POINT('Ctrl Pts',(-4.51835057975363,23.1218000776565,-1.4056613558427));
#4891=CARTESIAN_POINT('Ctrl Pts',(-3.67377298531822,23.2468000776565,-2.59934255826095));
#4892=CARTESIAN_POINT('Ctrl Pts',(-2.82919539088281,23.3718000776565,-3.79302376067921));
#4893=CARTESIAN_POINT('Ctrl Pts',(-1.44428955719605,23.4968000776565,-4.2623018848757));
#4894=CARTESIAN_POINT('Ctrl Pts',(-0.0593837235092896,23.6218000776565,
-4.7315800090722));
#4895=CARTESIAN_POINT('Ctrl Pts',(1.33686339217848,23.7468000776565,-4.29720676178068));
#4896=CARTESIAN_POINT('Ctrl Pts',(2.73311050786625,23.8718000776565,-3.86283351448915));
#4897=CARTESIAN_POINT('Ctrl Pts',(3.60737996405631,23.9968000776565,-2.69072471237131));
#4898=CARTESIAN_POINT('Ctrl Pts',(4.48164942024637,24.1218000776565,-1.51861591025346));
#4899=CARTESIAN_POINT('Ctrl Pts',(4.5,24.2468000776565,-0.0564772772053798));
#4900=CARTESIAN_POINT('Ctrl Pts',(4.51835057975363,24.3718000776565,1.4056613558427));
#4901=CARTESIAN_POINT('Ctrl Pts',(3.67377298531822,24.4968000776565,2.59934255826095));
#4902=CARTESIAN_POINT('Ctrl Pts',(2.82919539088281,24.6218000776565,3.7930237606792));
#4903=CARTESIAN_POINT('Ctrl Pts',(1.44428955719605,24.7468000776565,4.2623018848757));
#4904=CARTESIAN_POINT('Ctrl Pts',(0.0593837235092902,24.8718000776565,4.7315800090722));
#4905=CARTESIAN_POINT('Ctrl Pts',(-1.33686339217848,24.9968000776565,4.29720676178068));
#4906=CARTESIAN_POINT('Ctrl Pts',(-2.73311050786625,25.1218000776565,3.86283351448915));
#4907=CARTESIAN_POINT('Ctrl Pts',(-3.60737996405631,25.2468000776565,2.69072471237131));
#4908=CARTESIAN_POINT('Ctrl Pts',(-4.48164942024637,25.3718000776565,1.51861591025346));
#4909=CARTESIAN_POINT('Ctrl Pts',(-4.5,25.4968000776565,0.0564772772053793));
#4910=CARTESIAN_POINT('Ctrl Pts',(-4.51835057975363,25.6218000776565,-1.4056613558427));
#4911=CARTESIAN_POINT('Ctrl Pts',(-3.67377298531822,25.7468000776565,-2.59934255826095));
#4912=CARTESIAN_POINT('Ctrl Pts',(-2.82919539088281,25.8718000776565,-3.79302376067921));
#4913=CARTESIAN_POINT('Ctrl Pts',(-1.44428955719605,25.9968000776565,-4.2623018848757));
#4914=CARTESIAN_POINT('Ctrl Pts',(-0.0593837235092896,26.1218000776565,
-4.7315800090722));
#4915=CARTESIAN_POINT('Ctrl Pts',(1.33686339217848,26.2468000776565,-4.29720676178068));
#4916=CARTESIAN_POINT('Ctrl Pts',(2.73311050786625,26.3718000776565,-3.86283351448915));
#4917=CARTESIAN_POINT('Ctrl Pts',(3.60737996405631,26.4968000776565,-2.69072471237131));
#4918=CARTESIAN_POINT('Ctrl Pts',(4.48164942024637,26.6218000776565,-1.51861591025346));
#4919=CARTESIAN_POINT('Ctrl Pts',(4.5,26.7468000776565,-0.0564772772053798));
#4920=CARTESIAN_POINT('Ctrl Pts',(4.51835057975363,26.8718000776565,1.4056613558427));
#4921=CARTESIAN_POINT('Ctrl Pts',(3.67377298531822,26.9968000776565,2.59934255826095));
#4922=CARTESIAN_POINT('Ctrl Pts',(2.82919539088281,27.1218000776565,3.7930237606792));
#4923=CARTESIAN_POINT('Ctrl Pts',(1.44428955719605,27.2468000776565,4.2623018848757));
#4924=CARTESIAN_POINT('Ctrl Pts',(0.0593837235092902,27.3718000776565,4.7315800090722));
#4925=CARTESIAN_POINT('Ctrl Pts',(-1.33686339217848,27.4968000776565,4.29720676178068));
#4926=CARTESIAN_POINT('Ctrl Pts',(-2.73311050786625,27.6218000776565,3.86283351448915));
#4927=CARTESIAN_POINT('Ctrl Pts',(-3.60737996405631,27.7468000776565,2.69072471237131));
#4928=CARTESIAN_POINT('Ctrl Pts',(-4.48164942024637,27.8718000776565,1.51861591025346));
#4929=CARTESIAN_POINT('Ctrl Pts',(-4.5,27.9968000776565,0.0564772772053793));
#4930=CARTESIAN_POINT('Ctrl Pts',(-4.51835057975363,28.1218000776565,-1.4056613558427));
#4931=CARTESIAN_POINT('Ctrl Pts',(-3.67377298531822,28.2468000776565,-2.59934255826095));
#4932=CARTESIAN_POINT('Ctrl Pts',(-2.82919539088281,28.3718000776565,-3.79302376067921));
#4933=CARTESIAN_POINT('Ctrl Pts',(-1.44428955719605,28.4968000776565,-4.2623018848757));
#4934=CARTESIAN_POINT('Ctrl Pts',(-0.0593837235092896,28.6218000776565,
-4.7315800090722));
#4935=CARTESIAN_POINT('Ctrl Pts',(1.33686339217848,28.7468000776565,-4.29720676178068));
#4936=CARTESIAN_POINT('Ctrl Pts',(2.73311050786625,28.8718000776565,-3.86283351448915));
#4937=CARTESIAN_POINT('Ctrl Pts',(3.60737996405631,28.9968000776565,-2.69072471237131));
#4938=CARTESIAN_POINT('Ctrl Pts',(4.48164942024637,29.1218000776565,-1.51861591025346));
#4939=CARTESIAN_POINT('Ctrl Pts',(4.5,29.2468000776565,-0.0564772772053798));
#4940=CARTESIAN_POINT('Ctrl Pts',(4.51835057975363,29.3718000776565,1.4056613558427));
#4941=CARTESIAN_POINT('Ctrl Pts',(3.67377298531822,29.4968000776565,2.59934255826095));
#4942=CARTESIAN_POINT('Ctrl Pts',(2.82919539088281,29.6218000776565,3.7930237606792));
#4943=CARTESIAN_POINT('Ctrl Pts',(1.44428955719605,29.7468000776565,4.2623018848757));
#4944=CARTESIAN_POINT('Ctrl Pts',(0.0593837235092902,29.8718000776565,4.7315800090722));
#4945=CARTESIAN_POINT('Ctrl Pts',(-1.33686339217848,29.9968000776565,4.29720676178068));
#4946=CARTESIAN_POINT('Ctrl Pts',(-2.73311050786625,30.1218000776565,3.86283351448915));
#4947=CARTESIAN_POINT('Ctrl Pts',(-3.60737996405631,30.2468000776565,2.69072471237131));
#4948=CARTESIAN_POINT('Ctrl Pts',(-4.48164942024637,30.3718000776565,1.51861591025346));
#4949=CARTESIAN_POINT('Ctrl Pts',(-4.5,30.4968000776565,0.0564772772053793));
#4950=CARTESIAN_POINT('Ctrl Pts',(-4.51835057975363,30.6218000776565,-1.4056613558427));
#4951=CARTESIAN_POINT('Ctrl Pts',(-3.67377298531822,30.7468000776565,-2.59934255826095));
#4952=CARTESIAN_POINT('Ctrl Pts',(-2.82919539088281,30.8718000776565,-3.79302376067921));
#4953=CARTESIAN_POINT('Ctrl Pts',(-1.44428955719605,30.9968000776565,-4.2623018848757));
#4954=CARTESIAN_POINT('Ctrl Pts',(-0.0593837235092896,31.1218000776565,
-4.7315800090722));
#4955=CARTESIAN_POINT('Ctrl Pts',(1.33686339217848,31.2468000776565,-4.29720676178068));
#4956=CARTESIAN_POINT('Ctrl Pts',(2.73311050786625,31.3718000776565,-3.86283351448915));
#4957=CARTESIAN_POINT('Ctrl Pts',(3.60737996405631,31.4968000776565,-2.69072471237131));
#4958=CARTESIAN_POINT('Ctrl Pts',(4.48164942024637,31.6218000776565,-1.51861591025346));
#4959=CARTESIAN_POINT('Ctrl Pts',(4.5,31.7468000776565,-0.0564772772053798));
#4960=CARTESIAN_POINT('Ctrl Pts',(4.51835057975363,31.8718000776565,1.4056613558427));
#4961=CARTESIAN_POINT('Ctrl Pts',(3.67377298531822,31.9968000776565,2.59934255826095));
#4962=CARTESIAN_POINT('Ctrl Pts',(2.82919539088281,32.1218000776565,3.7930237606792));
#4963=CARTESIAN_POINT('Ctrl Pts',(1.44428955719605,32.2468000776565,4.2623018848757));
#4964=CARTESIAN_POINT('Ctrl Pts',(0.0593837235092902,32.3718000776565,4.7315800090722));
#4965=CARTESIAN_POINT('Ctrl Pts',(-1.33686339217848,32.4968000776565,4.29720676178068));
#4966=CARTESIAN_POINT('Ctrl Pts',(-2.73311050786625,32.6218000776565,3.86283351448915));
#4967=CARTESIAN_POINT('Ctrl Pts',(-3.60737996405631,32.7468000776565,2.69072471237131));
#4968=CARTESIAN_POINT('Ctrl Pts',(-4.48164942024637,32.8718000776565,1.51861591025346));
#4969=CARTESIAN_POINT('Ctrl Pts',(-4.5,32.9968000776565,0.0564772772053793));
#4970=CARTESIAN_POINT('Ctrl Pts',(-4.51835057975363,33.1218000776565,-1.4056613558427));
#4971=CARTESIAN_POINT('Ctrl Pts',(-3.67377298531822,33.2468000776565,-2.59934255826095));
#4972=CARTESIAN_POINT('Ctrl Pts',(-2.82919539088281,33.3718000776565,-3.79302376067921));
#4973=CARTESIAN_POINT('Ctrl Pts',(-1.44428955719605,33.4968000776565,-4.2623018848757));
#4974=CARTESIAN_POINT('Ctrl Pts',(-0.0593837235092896,33.6218000776565,
-4.7315800090722));
#4975=CARTESIAN_POINT('Ctrl Pts',(1.33686339217848,33.7468000776565,-4.29720676178068));
#4976=CARTESIAN_POINT('Ctrl Pts',(2.73311050786625,33.8718000776565,-3.86283351448915));
#4977=CARTESIAN_POINT('Ctrl Pts',(3.60737996405631,33.9968000776565,-2.69072471237131));
#4978=CARTESIAN_POINT('Ctrl Pts',(4.48164942024637,34.1218000776565,-1.51861591025346));
#4979=CARTESIAN_POINT('Ctrl Pts',(4.5,34.2468000776565,-0.0564772772053798));
#4980=CARTESIAN_POINT('Ctrl Pts',(4.51835057975363,34.3718000776565,1.4056613558427));
#4981=CARTESIAN_POINT('Ctrl Pts',(3.67377298531822,34.4968000776565,2.59934255826095));
#4982=CARTESIAN_POINT('Ctrl Pts',(2.82919539088281,34.6218000776565,3.7930237606792));
#4983=CARTESIAN_POINT('Ctrl Pts',(1.44428955719605,34.7468000776565,4.2623018848757));
#4984=CARTESIAN_POINT('Ctrl Pts',(0.0593837235092902,34.8718000776565,4.7315800090722));
#4985=CARTESIAN_POINT('Ctrl Pts',(-1.33686339217848,34.9968000776565,4.29720676178068));
#4986=CARTESIAN_POINT('Ctrl Pts',(-2.73311050786625,35.1218000776565,3.86283351448915));
#4987=CARTESIAN_POINT('Ctrl Pts',(-3.60737996405631,35.2468000776565,2.69072471237131));
#4988=CARTESIAN_POINT('Ctrl Pts',(-4.48164942024637,35.3718000776565,1.51861591025346));
#4989=CARTESIAN_POINT('Ctrl Pts',(-4.5,35.4968000776565,0.0564772772053793));
#4990=CARTESIAN_POINT('Ctrl Pts',(-4.51835057975363,35.6218000776565,-1.4056613558427));
#4991=CARTESIAN_POINT('Ctrl Pts',(-3.67377298531822,35.7468000776565,-2.59934255826095));
#4992=CARTESIAN_POINT('Ctrl Pts',(-2.82919539088281,35.8718000776565,-3.79302376067921));
#4993=CARTESIAN_POINT('Ctrl Pts',(-1.44428955719605,35.9968000776565,-4.2623018848757));
#4994=CARTESIAN_POINT('Ctrl Pts',(-0.0593837235092896,36.1218000776565,
-4.7315800090722));
#4995=CARTESIAN_POINT('Ctrl Pts',(1.33686339217848,36.2468000776565,-4.29720676178068));
#4996=CARTESIAN_POINT('Ctrl Pts',(2.73311050786625,36.3718000776565,-3.86283351448915));
#4997=CARTESIAN_POINT('Ctrl Pts',(3.60737996405631,36.4968000776565,-2.69072471237131));
#4998=CARTESIAN_POINT('Ctrl Pts',(4.48164942024637,36.6218000776565,-1.51861591025346));
#4999=CARTESIAN_POINT('Ctrl Pts',(4.5,36.7468000776565,-0.0564772772053798));
#5000=CARTESIAN_POINT('Ctrl Pts',(4.51835057975363,36.8718000776565,1.4056613558427));
#5001=CARTESIAN_POINT('Ctrl Pts',(3.67377298531822,36.9968000776565,2.59934255826095));
#5002=CARTESIAN_POINT('Ctrl Pts',(2.82919539088281,37.1218000776565,3.7930237606792));
#5003=CARTESIAN_POINT('Ctrl Pts',(1.44428955719605,37.2468000776565,4.2623018848757));
#5004=CARTESIAN_POINT('Ctrl Pts',(0.0593837235092902,37.3718000776565,4.7315800090722));
#5005=CARTESIAN_POINT('Ctrl Pts',(-1.33686339217848,37.4968000776565,4.29720676178068));
#5006=CARTESIAN_POINT('Ctrl Pts',(-2.73311050786625,37.6218000776565,3.86283351448915));
#5007=CARTESIAN_POINT('Ctrl Pts',(-3.60737996405631,37.7468000776565,2.69072471237131));
#5008=CARTESIAN_POINT('Ctrl Pts',(-4.48164942024637,37.8718000776565,1.51861591025346));
#5009=CARTESIAN_POINT('Ctrl Pts',(-4.5,37.9968000776565,0.0564772772053793));
#5010=CARTESIAN_POINT('Ctrl Pts',(-4.51835057975363,38.1218000776565,-1.4056613558427));
#5011=CARTESIAN_POINT('Ctrl Pts',(-3.67377298531822,38.2468000776565,-2.59934255826095));
#5012=CARTESIAN_POINT('Ctrl Pts',(-2.82919539088281,38.3718000776565,-3.79302376067921));
#5013=CARTESIAN_POINT('Ctrl Pts',(-1.44428955719605,38.4968000776565,-4.2623018848757));
#5014=CARTESIAN_POINT('Ctrl Pts',(-0.0593837235092896,38.6218000776565,
-4.7315800090722));
#5015=CARTESIAN_POINT('Ctrl Pts',(1.33686339217848,38.7468000776565,-4.29720676178068));
#5016=CARTESIAN_POINT('Ctrl Pts',(2.73311050786625,38.8718000776565,-3.86283351448915));
#5017=CARTESIAN_POINT('Ctrl Pts',(3.60737996405631,38.9968000776565,-2.69072471237131));
#5018=CARTESIAN_POINT('Ctrl Pts',(4.48164942024637,39.1218000776565,-1.51861591025346));
#5019=CARTESIAN_POINT('Ctrl Pts',(4.5,39.2468000776565,-0.0564772772053798));
#5020=CARTESIAN_POINT('Ctrl Pts',(4.51835057975363,39.3718000776565,1.4056613558427));
#5021=CARTESIAN_POINT('Ctrl Pts',(3.67377298531822,39.4968000776565,2.59934255826095));
#5022=CARTESIAN_POINT('Ctrl Pts',(2.82919539088281,39.6218000776565,3.7930237606792));
#5023=CARTESIAN_POINT('Ctrl Pts',(1.44428955719605,39.7468000776565,4.2623018848757));
#5024=CARTESIAN_POINT('Ctrl Pts',(0.0593837235092902,39.8718000776565,4.7315800090722));
#5025=CARTESIAN_POINT('Ctrl Pts',(-1.33686339217848,39.9968000776565,4.29720676178068));
#5026=CARTESIAN_POINT('Ctrl Pts',(-2.73311050786625,40.1218000776565,3.86283351448915));
#5027=CARTESIAN_POINT('Ctrl Pts',(-3.60737996405631,40.2468000776565,2.69072471237131));
#5028=CARTESIAN_POINT('Ctrl Pts',(-4.48164942024637,40.3718000776565,1.51861591025346));
#5029=CARTESIAN_POINT('Ctrl Pts',(-4.5,40.4968000776565,0.0564772772053793));
#5030=CARTESIAN_POINT('Ctrl Pts',(-3.5,15.4968000776565,0.0564772772053689));
#5031=CARTESIAN_POINT('Ctrl Pts',(-3.51835057975363,15.6218000776565,-1.0807416596098));
#5032=CARTESIAN_POINT('Ctrl Pts',(-2.86475599094327,15.7468000776565,-2.01155730596849));
#5033=CARTESIAN_POINT('Ctrl Pts',(-2.2111614021329,15.8718000776565,-2.94237295232717));
#5034=CARTESIAN_POINT('Ctrl Pts',(-1.13527256282109,15.9968000776565,-3.31124536858055));
#5035=CARTESIAN_POINT('Ctrl Pts',(-0.0593837235092786,16.1218000776565,
-3.68011778483394));
#5036=CARTESIAN_POINT('Ctrl Pts',(1.02784639780354,16.2468000776565,-3.34615024548552));
#5037=CARTESIAN_POINT('Ctrl Pts',(2.11507651911636,16.3718000776565,-3.01218270613711));
#5038=CARTESIAN_POINT('Ctrl Pts',(2.79836296968137,16.4968000776565,-2.10293946007882));
#5039=CARTESIAN_POINT('Ctrl Pts',(3.48164942024637,16.6218000776565,-1.19369621402054));
#5040=CARTESIAN_POINT('Ctrl Pts',(3.5,16.7468000776565,-0.0564772772053694));
#5041=CARTESIAN_POINT('Ctrl Pts',(3.51835057975363,16.8718000776565,1.0807416596098));
#5042=CARTESIAN_POINT('Ctrl Pts',(2.86475599094327,16.9968000776565,2.01155730596849));
#5043=CARTESIAN_POINT('Ctrl Pts',(2.2111614021329,17.1218000776565,2.94237295232717));
#5044=CARTESIAN_POINT('Ctrl Pts',(1.13527256282109,17.2468000776565,3.31124536858055));
#5045=CARTESIAN_POINT('Ctrl Pts',(0.0593837235092791,17.3718000776565,3.68011778483394));
#5046=CARTESIAN_POINT('Ctrl Pts',(-1.02784639780354,17.4968000776565,3.34615024548552));
#5047=CARTESIAN_POINT('Ctrl Pts',(-2.11507651911636,17.6218000776565,3.01218270613711));
#5048=CARTESIAN_POINT('Ctrl Pts',(-2.79836296968137,17.7468000776565,2.10293946007882));
#5049=CARTESIAN_POINT('Ctrl Pts',(-3.48164942024637,17.8718000776565,1.19369621402054));
#5050=CARTESIAN_POINT('Ctrl Pts',(-3.5,17.9968000776565,0.0564772772053689));
#5051=CARTESIAN_POINT('Ctrl Pts',(-3.51835057975363,18.1218000776565,-1.0807416596098));
#5052=CARTESIAN_POINT('Ctrl Pts',(-2.86475599094327,18.2468000776565,-2.01155730596849));
#5053=CARTESIAN_POINT('Ctrl Pts',(-2.2111614021329,18.3718000776565,-2.94237295232717));
#5054=CARTESIAN_POINT('Ctrl Pts',(-1.13527256282109,18.4968000776565,-3.31124536858055));
#5055=CARTESIAN_POINT('Ctrl Pts',(-0.0593837235092786,18.6218000776565,
-3.68011778483394));
#5056=CARTESIAN_POINT('Ctrl Pts',(1.02784639780354,18.7468000776565,-3.34615024548552));
#5057=CARTESIAN_POINT('Ctrl Pts',(2.11507651911636,18.8718000776565,-3.01218270613711));
#5058=CARTESIAN_POINT('Ctrl Pts',(2.79836296968137,18.9968000776565,-2.10293946007882));
#5059=CARTESIAN_POINT('Ctrl Pts',(3.48164942024637,19.1218000776565,-1.19369621402054));
#5060=CARTESIAN_POINT('Ctrl Pts',(3.5,19.2468000776565,-0.0564772772053694));
#5061=CARTESIAN_POINT('Ctrl Pts',(3.51835057975363,19.3718000776565,1.0807416596098));
#5062=CARTESIAN_POINT('Ctrl Pts',(2.86475599094327,19.4968000776565,2.01155730596849));
#5063=CARTESIAN_POINT('Ctrl Pts',(2.2111614021329,19.6218000776565,2.94237295232717));
#5064=CARTESIAN_POINT('Ctrl Pts',(1.13527256282109,19.7468000776565,3.31124536858055));
#5065=CARTESIAN_POINT('Ctrl Pts',(0.0593837235092791,19.8718000776565,3.68011778483394));
#5066=CARTESIAN_POINT('Ctrl Pts',(-1.02784639780354,19.9968000776565,3.34615024548552));
#5067=CARTESIAN_POINT('Ctrl Pts',(-2.11507651911636,20.1218000776565,3.01218270613711));
#5068=CARTESIAN_POINT('Ctrl Pts',(-2.79836296968137,20.2468000776565,2.10293946007882));
#5069=CARTESIAN_POINT('Ctrl Pts',(-3.48164942024637,20.3718000776565,1.19369621402054));
#5070=CARTESIAN_POINT('Ctrl Pts',(-3.5,20.4968000776565,0.0564772772053689));
#5071=CARTESIAN_POINT('Ctrl Pts',(-3.51835057975363,20.6218000776565,-1.0807416596098));
#5072=CARTESIAN_POINT('Ctrl Pts',(-2.86475599094327,20.7468000776565,-2.01155730596849));
#5073=CARTESIAN_POINT('Ctrl Pts',(-2.2111614021329,20.8718000776565,-2.94237295232717));
#5074=CARTESIAN_POINT('Ctrl Pts',(-1.13527256282109,20.9968000776565,-3.31124536858055));
#5075=CARTESIAN_POINT('Ctrl Pts',(-0.0593837235092786,21.1218000776565,
-3.68011778483394));
#5076=CARTESIAN_POINT('Ctrl Pts',(1.02784639780354,21.2468000776565,-3.34615024548552));
#5077=CARTESIAN_POINT('Ctrl Pts',(2.11507651911636,21.3718000776565,-3.01218270613711));
#5078=CARTESIAN_POINT('Ctrl Pts',(2.79836296968137,21.4968000776565,-2.10293946007882));
#5079=CARTESIAN_POINT('Ctrl Pts',(3.48164942024637,21.6218000776565,-1.19369621402054));
#5080=CARTESIAN_POINT('Ctrl Pts',(3.5,21.7468000776565,-0.0564772772053694));
#5081=CARTESIAN_POINT('Ctrl Pts',(3.51835057975363,21.8718000776565,1.0807416596098));
#5082=CARTESIAN_POINT('Ctrl Pts',(2.86475599094327,21.9968000776565,2.01155730596849));
#5083=CARTESIAN_POINT('Ctrl Pts',(2.2111614021329,22.1218000776565,2.94237295232717));
#5084=CARTESIAN_POINT('Ctrl Pts',(1.13527256282109,22.2468000776565,3.31124536858055));
#5085=CARTESIAN_POINT('Ctrl Pts',(0.0593837235092791,22.3718000776565,3.68011778483394));
#5086=CARTESIAN_POINT('Ctrl Pts',(-1.02784639780354,22.4968000776565,3.34615024548552));
#5087=CARTESIAN_POINT('Ctrl Pts',(-2.11507651911636,22.6218000776565,3.01218270613711));
#5088=CARTESIAN_POINT('Ctrl Pts',(-2.79836296968137,22.7468000776565,2.10293946007882));
#5089=CARTESIAN_POINT('Ctrl Pts',(-3.48164942024637,22.8718000776565,1.19369621402054));
#5090=CARTESIAN_POINT('Ctrl Pts',(-3.5,22.9968000776565,0.0564772772053689));
#5091=CARTESIAN_POINT('Ctrl Pts',(-3.51835057975363,23.1218000776565,-1.0807416596098));
#5092=CARTESIAN_POINT('Ctrl Pts',(-2.86475599094327,23.2468000776565,-2.01155730596849));
#5093=CARTESIAN_POINT('Ctrl Pts',(-2.2111614021329,23.3718000776565,-2.94237295232717));
#5094=CARTESIAN_POINT('Ctrl Pts',(-1.13527256282109,23.4968000776565,-3.31124536858055));
#5095=CARTESIAN_POINT('Ctrl Pts',(-0.0593837235092786,23.6218000776565,
-3.68011778483394));
#5096=CARTESIAN_POINT('Ctrl Pts',(1.02784639780354,23.7468000776565,-3.34615024548552));
#5097=CARTESIAN_POINT('Ctrl Pts',(2.11507651911636,23.8718000776565,-3.01218270613711));
#5098=CARTESIAN_POINT('Ctrl Pts',(2.79836296968137,23.9968000776565,-2.10293946007882));
#5099=CARTESIAN_POINT('Ctrl Pts',(3.48164942024637,24.1218000776565,-1.19369621402054));
#5100=CARTESIAN_POINT('Ctrl Pts',(3.5,24.2468000776565,-0.0564772772053694));
#5101=CARTESIAN_POINT('Ctrl Pts',(3.51835057975363,24.3718000776565,1.0807416596098));
#5102=CARTESIAN_POINT('Ctrl Pts',(2.86475599094327,24.4968000776565,2.01155730596849));
#5103=CARTESIAN_POINT('Ctrl Pts',(2.2111614021329,24.6218000776565,2.94237295232717));
#5104=CARTESIAN_POINT('Ctrl Pts',(1.13527256282109,24.7468000776565,3.31124536858055));
#5105=CARTESIAN_POINT('Ctrl Pts',(0.0593837235092791,24.8718000776565,3.68011778483394));
#5106=CARTESIAN_POINT('Ctrl Pts',(-1.02784639780354,24.9968000776565,3.34615024548552));
#5107=CARTESIAN_POINT('Ctrl Pts',(-2.11507651911636,25.1218000776565,3.01218270613711));
#5108=CARTESIAN_POINT('Ctrl Pts',(-2.79836296968137,25.2468000776565,2.10293946007882));
#5109=CARTESIAN_POINT('Ctrl Pts',(-3.48164942024637,25.3718000776565,1.19369621402054));
#5110=CARTESIAN_POINT('Ctrl Pts',(-3.5,25.4968000776565,0.0564772772053689));
#5111=CARTESIAN_POINT('Ctrl Pts',(-3.51835057975363,25.6218000776565,-1.0807416596098));
#5112=CARTESIAN_POINT('Ctrl Pts',(-2.86475599094327,25.7468000776565,-2.01155730596849));
#5113=CARTESIAN_POINT('Ctrl Pts',(-2.2111614021329,25.8718000776565,-2.94237295232717));
#5114=CARTESIAN_POINT('Ctrl Pts',(-1.13527256282109,25.9968000776565,-3.31124536858055));
#5115=CARTESIAN_POINT('Ctrl Pts',(-0.0593837235092786,26.1218000776565,
-3.68011778483394));
#5116=CARTESIAN_POINT('Ctrl Pts',(1.02784639780354,26.2468000776565,-3.34615024548552));
#5117=CARTESIAN_POINT('Ctrl Pts',(2.11507651911636,26.3718000776565,-3.01218270613711));
#5118=CARTESIAN_POINT('Ctrl Pts',(2.79836296968137,26.4968000776565,-2.10293946007882));
#5119=CARTESIAN_POINT('Ctrl Pts',(3.48164942024637,26.6218000776565,-1.19369621402054));
#5120=CARTESIAN_POINT('Ctrl Pts',(3.5,26.7468000776565,-0.0564772772053694));
#5121=CARTESIAN_POINT('Ctrl Pts',(3.51835057975363,26.8718000776565,1.0807416596098));
#5122=CARTESIAN_POINT('Ctrl Pts',(2.86475599094327,26.9968000776565,2.01155730596849));
#5123=CARTESIAN_POINT('Ctrl Pts',(2.2111614021329,27.1218000776565,2.94237295232717));
#5124=CARTESIAN_POINT('Ctrl Pts',(1.13527256282109,27.2468000776565,3.31124536858055));
#5125=CARTESIAN_POINT('Ctrl Pts',(0.0593837235092791,27.3718000776565,3.68011778483394));
#5126=CARTESIAN_POINT('Ctrl Pts',(-1.02784639780354,27.4968000776565,3.34615024548552));
#5127=CARTESIAN_POINT('Ctrl Pts',(-2.11507651911636,27.6218000776565,3.01218270613711));
#5128=CARTESIAN_POINT('Ctrl Pts',(-2.79836296968137,27.7468000776565,2.10293946007882));
#5129=CARTESIAN_POINT('Ctrl Pts',(-3.48164942024637,27.8718000776565,1.19369621402054));
#5130=CARTESIAN_POINT('Ctrl Pts',(-3.5,27.9968000776565,0.0564772772053689));
#5131=CARTESIAN_POINT('Ctrl Pts',(-3.51835057975363,28.1218000776565,-1.0807416596098));
#5132=CARTESIAN_POINT('Ctrl Pts',(-2.86475599094327,28.2468000776565,-2.01155730596849));
#5133=CARTESIAN_POINT('Ctrl Pts',(-2.2111614021329,28.3718000776565,-2.94237295232717));
#5134=CARTESIAN_POINT('Ctrl Pts',(-1.13527256282109,28.4968000776565,-3.31124536858055));
#5135=CARTESIAN_POINT('Ctrl Pts',(-0.0593837235092786,28.6218000776565,
-3.68011778483394));
#5136=CARTESIAN_POINT('Ctrl Pts',(1.02784639780354,28.7468000776565,-3.34615024548552));
#5137=CARTESIAN_POINT('Ctrl Pts',(2.11507651911636,28.8718000776565,-3.01218270613711));
#5138=CARTESIAN_POINT('Ctrl Pts',(2.79836296968137,28.9968000776565,-2.10293946007882));
#5139=CARTESIAN_POINT('Ctrl Pts',(3.48164942024637,29.1218000776565,-1.19369621402054));
#5140=CARTESIAN_POINT('Ctrl Pts',(3.5,29.2468000776565,-0.0564772772053694));
#5141=CARTESIAN_POINT('Ctrl Pts',(3.51835057975363,29.3718000776565,1.0807416596098));
#5142=CARTESIAN_POINT('Ctrl Pts',(2.86475599094327,29.4968000776565,2.01155730596849));
#5143=CARTESIAN_POINT('Ctrl Pts',(2.2111614021329,29.6218000776565,2.94237295232717));
#5144=CARTESIAN_POINT('Ctrl Pts',(1.13527256282109,29.7468000776565,3.31124536858055));
#5145=CARTESIAN_POINT('Ctrl Pts',(0.0593837235092791,29.8718000776565,3.68011778483394));
#5146=CARTESIAN_POINT('Ctrl Pts',(-1.02784639780354,29.9968000776565,3.34615024548552));
#5147=CARTESIAN_POINT('Ctrl Pts',(-2.11507651911636,30.1218000776565,3.01218270613711));
#5148=CARTESIAN_POINT('Ctrl Pts',(-2.79836296968137,30.2468000776565,2.10293946007882));
#5149=CARTESIAN_POINT('Ctrl Pts',(-3.48164942024637,30.3718000776565,1.19369621402054));
#5150=CARTESIAN_POINT('Ctrl Pts',(-3.5,30.4968000776565,0.0564772772053689));
#5151=CARTESIAN_POINT('Ctrl Pts',(-3.51835057975363,30.6218000776565,-1.0807416596098));
#5152=CARTESIAN_POINT('Ctrl Pts',(-2.86475599094327,30.7468000776565,-2.01155730596849));
#5153=CARTESIAN_POINT('Ctrl Pts',(-2.2111614021329,30.8718000776565,-2.94237295232717));
#5154=CARTESIAN_POINT('Ctrl Pts',(-1.13527256282109,30.9968000776565,-3.31124536858055));
#5155=CARTESIAN_POINT('Ctrl Pts',(-0.0593837235092786,31.1218000776565,
-3.68011778483394));
#5156=CARTESIAN_POINT('Ctrl Pts',(1.02784639780354,31.2468000776565,-3.34615024548552));
#5157=CARTESIAN_POINT('Ctrl Pts',(2.11507651911636,31.3718000776565,-3.01218270613711));
#5158=CARTESIAN_POINT('Ctrl Pts',(2.79836296968137,31.4968000776565,-2.10293946007882));
#5159=CARTESIAN_POINT('Ctrl Pts',(3.48164942024637,31.6218000776565,-1.19369621402054));
#5160=CARTESIAN_POINT('Ctrl Pts',(3.5,31.7468000776565,-0.0564772772053694));
#5161=CARTESIAN_POINT('Ctrl Pts',(3.51835057975363,31.8718000776565,1.0807416596098));
#5162=CARTESIAN_POINT('Ctrl Pts',(2.86475599094327,31.9968000776565,2.01155730596849));
#5163=CARTESIAN_POINT('Ctrl Pts',(2.2111614021329,32.1218000776565,2.94237295232717));
#5164=CARTESIAN_POINT('Ctrl Pts',(1.13527256282109,32.2468000776565,3.31124536858055));
#5165=CARTESIAN_POINT('Ctrl Pts',(0.0593837235092791,32.3718000776565,3.68011778483394));
#5166=CARTESIAN_POINT('Ctrl Pts',(-1.02784639780354,32.4968000776565,3.34615024548552));
#5167=CARTESIAN_POINT('Ctrl Pts',(-2.11507651911636,32.6218000776565,3.01218270613711));
#5168=CARTESIAN_POINT('Ctrl Pts',(-2.79836296968137,32.7468000776565,2.10293946007882));
#5169=CARTESIAN_POINT('Ctrl Pts',(-3.48164942024637,32.8718000776565,1.19369621402054));
#5170=CARTESIAN_POINT('Ctrl Pts',(-3.5,32.9968000776565,0.0564772772053689));
#5171=CARTESIAN_POINT('Ctrl Pts',(-3.51835057975363,33.1218000776565,-1.0807416596098));
#5172=CARTESIAN_POINT('Ctrl Pts',(-2.86475599094327,33.2468000776565,-2.01155730596849));
#5173=CARTESIAN_POINT('Ctrl Pts',(-2.2111614021329,33.3718000776565,-2.94237295232717));
#5174=CARTESIAN_POINT('Ctrl Pts',(-1.13527256282109,33.4968000776565,-3.31124536858055));
#5175=CARTESIAN_POINT('Ctrl Pts',(-0.0593837235092786,33.6218000776565,
-3.68011778483394));
#5176=CARTESIAN_POINT('Ctrl Pts',(1.02784639780354,33.7468000776565,-3.34615024548552));
#5177=CARTESIAN_POINT('Ctrl Pts',(2.11507651911636,33.8718000776565,-3.01218270613711));
#5178=CARTESIAN_POINT('Ctrl Pts',(2.79836296968137,33.9968000776565,-2.10293946007882));
#5179=CARTESIAN_POINT('Ctrl Pts',(3.48164942024637,34.1218000776565,-1.19369621402054));
#5180=CARTESIAN_POINT('Ctrl Pts',(3.5,34.2468000776565,-0.0564772772053694));
#5181=CARTESIAN_POINT('Ctrl Pts',(3.51835057975363,34.3718000776565,1.0807416596098));
#5182=CARTESIAN_POINT('Ctrl Pts',(2.86475599094327,34.4968000776565,2.01155730596849));
#5183=CARTESIAN_POINT('Ctrl Pts',(2.2111614021329,34.6218000776565,2.94237295232717));
#5184=CARTESIAN_POINT('Ctrl Pts',(1.13527256282109,34.7468000776565,3.31124536858055));
#5185=CARTESIAN_POINT('Ctrl Pts',(0.0593837235092791,34.8718000776565,3.68011778483394));
#5186=CARTESIAN_POINT('Ctrl Pts',(-1.02784639780354,34.9968000776565,3.34615024548552));
#5187=CARTESIAN_POINT('Ctrl Pts',(-2.11507651911636,35.1218000776565,3.01218270613711));
#5188=CARTESIAN_POINT('Ctrl Pts',(-2.79836296968137,35.2468000776565,2.10293946007882));
#5189=CARTESIAN_POINT('Ctrl Pts',(-3.48164942024637,35.3718000776565,1.19369621402054));
#5190=CARTESIAN_POINT('Ctrl Pts',(-3.5,35.4968000776565,0.0564772772053689));
#5191=CARTESIAN_POINT('Ctrl Pts',(-3.51835057975363,35.6218000776565,-1.0807416596098));
#5192=CARTESIAN_POINT('Ctrl Pts',(-2.86475599094327,35.7468000776565,-2.01155730596849));
#5193=CARTESIAN_POINT('Ctrl Pts',(-2.2111614021329,35.8718000776565,-2.94237295232717));
#5194=CARTESIAN_POINT('Ctrl Pts',(-1.13527256282109,35.9968000776565,-3.31124536858055));
#5195=CARTESIAN_POINT('Ctrl Pts',(-0.0593837235092786,36.1218000776565,
-3.68011778483394));
#5196=CARTESIAN_POINT('Ctrl Pts',(1.02784639780354,36.2468000776565,-3.34615024548552));
#5197=CARTESIAN_POINT('Ctrl Pts',(2.11507651911636,36.3718000776565,-3.01218270613711));
#5198=CARTESIAN_POINT('Ctrl Pts',(2.79836296968137,36.4968000776565,-2.10293946007882));
#5199=CARTESIAN_POINT('Ctrl Pts',(3.48164942024637,36.6218000776565,-1.19369621402054));
#5200=CARTESIAN_POINT('Ctrl Pts',(3.5,36.7468000776565,-0.0564772772053694));
#5201=CARTESIAN_POINT('Ctrl Pts',(3.51835057975363,36.8718000776565,1.0807416596098));
#5202=CARTESIAN_POINT('Ctrl Pts',(2.86475599094327,36.9968000776565,2.01155730596849));
#5203=CARTESIAN_POINT('Ctrl Pts',(2.2111614021329,37.1218000776565,2.94237295232717));
#5204=CARTESIAN_POINT('Ctrl Pts',(1.13527256282109,37.2468000776565,3.31124536858055));
#5205=CARTESIAN_POINT('Ctrl Pts',(0.0593837235092791,37.3718000776565,3.68011778483394));
#5206=CARTESIAN_POINT('Ctrl Pts',(-1.02784639780354,37.4968000776565,3.34615024548552));
#5207=CARTESIAN_POINT('Ctrl Pts',(-2.11507651911636,37.6218000776565,3.01218270613711));
#5208=CARTESIAN_POINT('Ctrl Pts',(-2.79836296968137,37.7468000776565,2.10293946007882));
#5209=CARTESIAN_POINT('Ctrl Pts',(-3.48164942024637,37.8718000776565,1.19369621402054));
#5210=CARTESIAN_POINT('Ctrl Pts',(-3.5,37.9968000776565,0.0564772772053689));
#5211=CARTESIAN_POINT('Ctrl Pts',(-3.51835057975363,38.1218000776565,-1.0807416596098));
#5212=CARTESIAN_POINT('Ctrl Pts',(-2.86475599094327,38.2468000776565,-2.01155730596849));
#5213=CARTESIAN_POINT('Ctrl Pts',(-2.2111614021329,38.3718000776565,-2.94237295232717));
#5214=CARTESIAN_POINT('Ctrl Pts',(-1.13527256282109,38.4968000776565,-3.31124536858055));
#5215=CARTESIAN_POINT('Ctrl Pts',(-0.0593837235092786,38.6218000776565,
-3.68011778483394));
#5216=CARTESIAN_POINT('Ctrl Pts',(1.02784639780354,38.7468000776565,-3.34615024548552));
#5217=CARTESIAN_POINT('Ctrl Pts',(2.11507651911636,38.8718000776565,-3.01218270613711));
#5218=CARTESIAN_POINT('Ctrl Pts',(2.79836296968137,38.9968000776565,-2.10293946007882));
#5219=CARTESIAN_POINT('Ctrl Pts',(3.48164942024637,39.1218000776565,-1.19369621402054));
#5220=CARTESIAN_POINT('Ctrl Pts',(3.5,39.2468000776565,-0.0564772772053694));
#5221=CARTESIAN_POINT('Ctrl Pts',(3.51835057975363,39.3718000776565,1.0807416596098));
#5222=CARTESIAN_POINT('Ctrl Pts',(2.86475599094327,39.4968000776565,2.01155730596849));
#5223=CARTESIAN_POINT('Ctrl Pts',(2.2111614021329,39.6218000776565,2.94237295232717));
#5224=CARTESIAN_POINT('Ctrl Pts',(1.13527256282109,39.7468000776565,3.31124536858055));
#5225=CARTESIAN_POINT('Ctrl Pts',(0.0593837235092791,39.8718000776565,3.68011778483394));
#5226=CARTESIAN_POINT('Ctrl Pts',(-1.02784639780354,39.9968000776565,3.34615024548552));
#5227=CARTESIAN_POINT('Ctrl Pts',(-2.11507651911636,40.1218000776565,3.01218270613711));
#5228=CARTESIAN_POINT('Ctrl Pts',(-2.79836296968137,40.2468000776565,2.10293946007882));
#5229=CARTESIAN_POINT('Ctrl Pts',(-3.48164942024637,40.3718000776565,1.19369621402054));
#5230=CARTESIAN_POINT('Ctrl Pts',(-3.5,40.4968000776565,0.0564772772053689));
#5231=CARTESIAN_POINT('',(-1.05560584366888,15.,-3.33749696414134));
#5232=CARTESIAN_POINT('',(-3.,15.,3.04863211306834E-14));
#5233=CARTESIAN_POINT('Ctrl Pts',(-1.05560584366887,15.,-3.33749696414134));
#5234=CARTESIAN_POINT('Ctrl Pts',(-1.05394151307971,15.,-3.3325158524897));
#5235=CARTESIAN_POINT('Ctrl Pts',(-1.05302581964714,15.,-3.32739803279745));
#5236=CARTESIAN_POINT('Ctrl Pts',(-1.05250282072891,15.,-3.31638533458449));
#5237=CARTESIAN_POINT('Ctrl Pts',(-1.0530441514054,14.9999999999996,-3.31062365811979));
#5238=CARTESIAN_POINT('Ctrl Pts',(-1.05686193571968,14.9999999999996,-3.29147078572532));
#5239=CARTESIAN_POINT('Ctrl Pts',(-1.06302909045672,15.,-3.27779288376222));
#5240=CARTESIAN_POINT('Ctrl Pts',(-1.09049428069001,15.,-3.23176963091457));
#5241=CARTESIAN_POINT('Ctrl Pts',(-1.12473174639127,15.,-3.19498750811399));
#5242=CARTESIAN_POINT('Ctrl Pts',(-1.27982154446677,15.,-3.05221474570734));
#5243=CARTESIAN_POINT('Ctrl Pts',(-1.45769115884876,15.,-2.92194246708069));
#5244=CARTESIAN_POINT('Ctrl Pts',(-1.88593610007892,15.,-2.54883289900392));
#5245=CARTESIAN_POINT('Ctrl Pts',(-2.1703656445531,15.,-2.27198918349741));
#5246=CARTESIAN_POINT('Ctrl Pts',(-2.5725161275751,15.,-1.66624001122359));
#5247=CARTESIAN_POINT('Ctrl Pts',(-2.72305386070332,15.,-1.38777729550143));
#5248=CARTESIAN_POINT('Ctrl Pts',(-2.94442189004107,15.,-0.700038275746447));
#5249=CARTESIAN_POINT('Ctrl Pts',(-3.00000000000001,15.,-0.351019517027752));
#5250=CARTESIAN_POINT('Ctrl Pts',(-3.,15.,2.96464242044436E-14));
#5251=CARTESIAN_POINT('',(-3.5,39.5031999223435,-0.056477277205296));
#5252=CARTESIAN_POINT('Ctrl Pts',(-1.05560584366888,15.,-3.33749696414134));
#5253=CARTESIAN_POINT('Ctrl Pts',(-1.04174409073731,15.0016020898492,-3.34188125199396));
#5254=CARTESIAN_POINT('Ctrl Pts',(-1.02784639780361,15.0031999223435,-3.3461502454855));
#5255=CARTESIAN_POINT('Ctrl Pts',(0.0593837235092011,15.1281999223435,-3.68011778483394));
#5256=CARTESIAN_POINT('Ctrl Pts',(1.13527256282102,15.2531999223435,-3.31124536858058));
#5257=CARTESIAN_POINT('Ctrl Pts',(2.21116140213284,15.3781999223435,-2.94237295232722));
#5258=CARTESIAN_POINT('Ctrl Pts',(2.86475599094322,15.5031999223435,-2.01155730596855));
#5259=CARTESIAN_POINT('Ctrl Pts',(3.51835057975361,15.6281999223435,-1.08074165960988));
#5260=CARTESIAN_POINT('Ctrl Pts',(3.5,15.7531999223435,0.0564772772052952));
#5261=CARTESIAN_POINT('Ctrl Pts',(3.4816494202464,15.8781999223435,1.19369621402047));
#5262=CARTESIAN_POINT('Ctrl Pts',(2.79836296968141,16.0031999223435,2.10293946007876));
#5263=CARTESIAN_POINT('Ctrl Pts',(2.11507651911643,16.1281999223435,3.01218270613706));
#5264=CARTESIAN_POINT('Ctrl Pts',(1.02784639780361,16.2531999223435,3.3461502454855));
#5265=CARTESIAN_POINT('Ctrl Pts',(-0.0593837235092006,16.3781999223435,
3.68011778483394));
#5266=CARTESIAN_POINT('Ctrl Pts',(-1.13527256282102,16.5031999223435,3.31124536858058));
#5267=CARTESIAN_POINT('Ctrl Pts',(-2.21116140213284,16.6281999223435,2.94237295232722));
#5268=CARTESIAN_POINT('Ctrl Pts',(-2.86475599094322,16.7531999223435,2.01155730596855));
#5269=CARTESIAN_POINT('Ctrl Pts',(-3.51835057975361,16.8781999223435,1.08074165960988));
#5270=CARTESIAN_POINT('Ctrl Pts',(-3.5,17.0031999223435,-0.0564772772052956));
#5271=CARTESIAN_POINT('Ctrl Pts',(-3.4816494202464,17.1281999223435,-1.19369621402047));
#5272=CARTESIAN_POINT('Ctrl Pts',(-2.79836296968141,17.2531999223435,-2.10293946007877));
#5273=CARTESIAN_POINT('Ctrl Pts',(-2.11507651911643,17.3781999223435,-3.01218270613706));
#5274=CARTESIAN_POINT('Ctrl Pts',(-1.02784639780361,17.5031999223435,-3.3461502454855));
#5275=CARTESIAN_POINT('Ctrl Pts',(0.0593837235092011,17.6281999223435,-3.68011778483394));
#5276=CARTESIAN_POINT('Ctrl Pts',(1.13527256282102,17.7531999223435,-3.31124536858058));
#5277=CARTESIAN_POINT('Ctrl Pts',(2.21116140213284,17.8781999223435,-2.94237295232722));
#5278=CARTESIAN_POINT('Ctrl Pts',(2.86475599094322,18.0031999223435,-2.01155730596855));
#5279=CARTESIAN_POINT('Ctrl Pts',(3.51835057975361,18.1281999223435,-1.08074165960988));
#5280=CARTESIAN_POINT('Ctrl Pts',(3.5,18.2531999223435,0.0564772772052952));
#5281=CARTESIAN_POINT('Ctrl Pts',(3.4816494202464,18.3781999223435,1.19369621402047));
#5282=CARTESIAN_POINT('Ctrl Pts',(2.79836296968141,18.5031999223435,2.10293946007876));
#5283=CARTESIAN_POINT('Ctrl Pts',(2.11507651911643,18.6281999223435,3.01218270613706));
#5284=CARTESIAN_POINT('Ctrl Pts',(1.02784639780361,18.7531999223435,3.3461502454855));
#5285=CARTESIAN_POINT('Ctrl Pts',(-0.0593837235092006,18.8781999223435,
3.68011778483394));
#5286=CARTESIAN_POINT('Ctrl Pts',(-1.13527256282102,19.0031999223435,3.31124536858058));
#5287=CARTESIAN_POINT('Ctrl Pts',(-2.21116140213284,19.1281999223435,2.94237295232722));
#5288=CARTESIAN_POINT('Ctrl Pts',(-2.86475599094322,19.2531999223435,2.01155730596855));
#5289=CARTESIAN_POINT('Ctrl Pts',(-3.51835057975361,19.3781999223435,1.08074165960988));
#5290=CARTESIAN_POINT('Ctrl Pts',(-3.5,19.5031999223435,-0.0564772772052956));
#5291=CARTESIAN_POINT('Ctrl Pts',(-3.4816494202464,19.6281999223435,-1.19369621402047));
#5292=CARTESIAN_POINT('Ctrl Pts',(-2.79836296968141,19.7531999223435,-2.10293946007877));
#5293=CARTESIAN_POINT('Ctrl Pts',(-2.11507651911643,19.8781999223435,-3.01218270613706));
#5294=CARTESIAN_POINT('Ctrl Pts',(-1.02784639780361,20.0031999223435,-3.3461502454855));
#5295=CARTESIAN_POINT('Ctrl Pts',(0.0593837235092011,20.1281999223435,-3.68011778483394));
#5296=CARTESIAN_POINT('Ctrl Pts',(1.13527256282102,20.2531999223435,-3.31124536858058));
#5297=CARTESIAN_POINT('Ctrl Pts',(2.21116140213284,20.3781999223435,-2.94237295232722));
#5298=CARTESIAN_POINT('Ctrl Pts',(2.86475599094322,20.5031999223435,-2.01155730596855));
#5299=CARTESIAN_POINT('Ctrl Pts',(3.51835057975361,20.6281999223435,-1.08074165960988));
#5300=CARTESIAN_POINT('Ctrl Pts',(3.5,20.7531999223435,0.0564772772052952));
#5301=CARTESIAN_POINT('Ctrl Pts',(3.4816494202464,20.8781999223435,1.19369621402047));
#5302=CARTESIAN_POINT('Ctrl Pts',(2.79836296968141,21.0031999223435,2.10293946007876));
#5303=CARTESIAN_POINT('Ctrl Pts',(2.11507651911643,21.1281999223435,3.01218270613706));
#5304=CARTESIAN_POINT('Ctrl Pts',(1.02784639780361,21.2531999223435,3.3461502454855));
#5305=CARTESIAN_POINT('Ctrl Pts',(-0.0593837235092006,21.3781999223435,
3.68011778483394));
#5306=CARTESIAN_POINT('Ctrl Pts',(-1.13527256282102,21.5031999223435,3.31124536858058));
#5307=CARTESIAN_POINT('Ctrl Pts',(-2.21116140213284,21.6281999223435,2.94237295232722));
#5308=CARTESIAN_POINT('Ctrl Pts',(-2.86475599094322,21.7531999223435,2.01155730596855));
#5309=CARTESIAN_POINT('Ctrl Pts',(-3.51835057975361,21.8781999223435,1.08074165960988));
#5310=CARTESIAN_POINT('Ctrl Pts',(-3.5,22.0031999223435,-0.0564772772052956));
#5311=CARTESIAN_POINT('Ctrl Pts',(-3.4816494202464,22.1281999223435,-1.19369621402047));
#5312=CARTESIAN_POINT('Ctrl Pts',(-2.79836296968141,22.2531999223435,-2.10293946007877));
#5313=CARTESIAN_POINT('Ctrl Pts',(-2.11507651911643,22.3781999223435,-3.01218270613706));
#5314=CARTESIAN_POINT('Ctrl Pts',(-1.02784639780361,22.5031999223435,-3.3461502454855));
#5315=CARTESIAN_POINT('Ctrl Pts',(0.0593837235092011,22.6281999223435,-3.68011778483394));
#5316=CARTESIAN_POINT('Ctrl Pts',(1.13527256282102,22.7531999223435,-3.31124536858058));
#5317=CARTESIAN_POINT('Ctrl Pts',(2.21116140213284,22.8781999223435,-2.94237295232722));
#5318=CARTESIAN_POINT('Ctrl Pts',(2.86475599094322,23.0031999223435,-2.01155730596855));
#5319=CARTESIAN_POINT('Ctrl Pts',(3.51835057975361,23.1281999223435,-1.08074165960988));
#5320=CARTESIAN_POINT('Ctrl Pts',(3.5,23.2531999223435,0.0564772772052952));
#5321=CARTESIAN_POINT('Ctrl Pts',(3.4816494202464,23.3781999223435,1.19369621402047));
#5322=CARTESIAN_POINT('Ctrl Pts',(2.79836296968141,23.5031999223435,2.10293946007876));
#5323=CARTESIAN_POINT('Ctrl Pts',(2.11507651911643,23.6281999223435,3.01218270613706));
#5324=CARTESIAN_POINT('Ctrl Pts',(1.02784639780361,23.7531999223435,3.3461502454855));
#5325=CARTESIAN_POINT('Ctrl Pts',(-0.0593837235092006,23.8781999223435,
3.68011778483394));
#5326=CARTESIAN_POINT('Ctrl Pts',(-1.13527256282102,24.0031999223435,3.31124536858058));
#5327=CARTESIAN_POINT('Ctrl Pts',(-2.21116140213284,24.1281999223435,2.94237295232722));
#5328=CARTESIAN_POINT('Ctrl Pts',(-2.86475599094322,24.2531999223435,2.01155730596855));
#5329=CARTESIAN_POINT('Ctrl Pts',(-3.51835057975361,24.3781999223435,1.08074165960988));
#5330=CARTESIAN_POINT('Ctrl Pts',(-3.5,24.5031999223435,-0.0564772772052956));
#5331=CARTESIAN_POINT('Ctrl Pts',(-3.4816494202464,24.6281999223435,-1.19369621402047));
#5332=CARTESIAN_POINT('Ctrl Pts',(-2.79836296968141,24.7531999223435,-2.10293946007877));
#5333=CARTESIAN_POINT('Ctrl Pts',(-2.11507651911643,24.8781999223435,-3.01218270613706));
#5334=CARTESIAN_POINT('Ctrl Pts',(-1.02784639780361,25.0031999223435,-3.3461502454855));
#5335=CARTESIAN_POINT('Ctrl Pts',(0.0593837235092011,25.1281999223435,-3.68011778483394));
#5336=CARTESIAN_POINT('Ctrl Pts',(1.13527256282102,25.2531999223435,-3.31124536858058));
#5337=CARTESIAN_POINT('Ctrl Pts',(2.21116140213284,25.3781999223435,-2.94237295232722));
#5338=CARTESIAN_POINT('Ctrl Pts',(2.86475599094322,25.5031999223436,-2.01155730596855));
#5339=CARTESIAN_POINT('Ctrl Pts',(3.51835057975361,25.6281999223435,-1.08074165960988));
#5340=CARTESIAN_POINT('Ctrl Pts',(3.5,25.7531999223436,0.0564772772052952));
#5341=CARTESIAN_POINT('Ctrl Pts',(3.4816494202464,25.8781999223435,1.19369621402047));
#5342=CARTESIAN_POINT('Ctrl Pts',(2.79836296968141,26.0031999223435,2.10293946007876));
#5343=CARTESIAN_POINT('Ctrl Pts',(2.11507651911643,26.1281999223436,3.01218270613706));
#5344=CARTESIAN_POINT('Ctrl Pts',(1.02784639780361,26.2531999223435,3.3461502454855));
#5345=CARTESIAN_POINT('Ctrl Pts',(-0.0593837235092006,26.3781999223435,
3.68011778483394));
#5346=CARTESIAN_POINT('Ctrl Pts',(-1.13527256282102,26.5031999223435,3.31124536858058));
#5347=CARTESIAN_POINT('Ctrl Pts',(-2.21116140213284,26.6281999223435,2.94237295232722));
#5348=CARTESIAN_POINT('Ctrl Pts',(-2.86475599094322,26.7531999223436,2.01155730596855));
#5349=CARTESIAN_POINT('Ctrl Pts',(-3.51835057975361,26.8781999223435,1.08074165960988));
#5350=CARTESIAN_POINT('Ctrl Pts',(-3.5,27.0031999223436,-0.0564772772052956));
#5351=CARTESIAN_POINT('Ctrl Pts',(-3.4816494202464,27.1281999223435,-1.19369621402047));
#5352=CARTESIAN_POINT('Ctrl Pts',(-2.79836296968141,27.2531999223435,-2.10293946007877));
#5353=CARTESIAN_POINT('Ctrl Pts',(-2.11507651911643,27.3781999223436,-3.01218270613706));
#5354=CARTESIAN_POINT('Ctrl Pts',(-1.02784639780361,27.5031999223435,-3.3461502454855));
#5355=CARTESIAN_POINT('Ctrl Pts',(0.0593837235092011,27.6281999223435,-3.68011778483394));
#5356=CARTESIAN_POINT('Ctrl Pts',(1.13527256282102,27.7531999223435,-3.31124536858058));
#5357=CARTESIAN_POINT('Ctrl Pts',(2.21116140213284,27.8781999223435,-2.94237295232722));
#5358=CARTESIAN_POINT('Ctrl Pts',(2.86475599094322,28.0031999223435,-2.01155730596855));
#5359=CARTESIAN_POINT('Ctrl Pts',(3.51835057975361,28.1281999223435,-1.08074165960988));
#5360=CARTESIAN_POINT('Ctrl Pts',(3.5,28.2531999223435,0.0564772772052952));
#5361=CARTESIAN_POINT('Ctrl Pts',(3.4816494202464,28.3781999223435,1.19369621402047));
#5362=CARTESIAN_POINT('Ctrl Pts',(2.79836296968141,28.5031999223435,2.10293946007876));
#5363=CARTESIAN_POINT('Ctrl Pts',(2.11507651911643,28.6281999223435,3.01218270613706));
#5364=CARTESIAN_POINT('Ctrl Pts',(1.02784639780361,28.7531999223435,3.3461502454855));
#5365=CARTESIAN_POINT('Ctrl Pts',(-0.0593837235092006,28.8781999223435,
3.68011778483394));
#5366=CARTESIAN_POINT('Ctrl Pts',(-1.13527256282102,29.0031999223435,3.31124536858058));
#5367=CARTESIAN_POINT('Ctrl Pts',(-2.21116140213284,29.1281999223435,2.94237295232722));
#5368=CARTESIAN_POINT('Ctrl Pts',(-2.86475599094322,29.2531999223435,2.01155730596855));
#5369=CARTESIAN_POINT('Ctrl Pts',(-3.51835057975361,29.3781999223435,1.08074165960988));
#5370=CARTESIAN_POINT('Ctrl Pts',(-3.5,29.5031999223435,-0.0564772772052956));
#5371=CARTESIAN_POINT('Ctrl Pts',(-3.4816494202464,29.6281999223435,-1.19369621402047));
#5372=CARTESIAN_POINT('Ctrl Pts',(-2.79836296968141,29.7531999223435,-2.10293946007877));
#5373=CARTESIAN_POINT('Ctrl Pts',(-2.11507651911643,29.8781999223435,-3.01218270613706));
#5374=CARTESIAN_POINT('Ctrl Pts',(-1.02784639780361,30.0031999223435,-3.3461502454855));
#5375=CARTESIAN_POINT('Ctrl Pts',(0.0593837235092011,30.1281999223435,-3.68011778483394));
#5376=CARTESIAN_POINT('Ctrl Pts',(1.13527256282102,30.2531999223435,-3.31124536858058));
#5377=CARTESIAN_POINT('Ctrl Pts',(2.21116140213284,30.3781999223435,-2.94237295232722));
#5378=CARTESIAN_POINT('Ctrl Pts',(2.86475599094322,30.5031999223435,-2.01155730596855));
#5379=CARTESIAN_POINT('Ctrl Pts',(3.51835057975361,30.6281999223435,-1.08074165960988));
#5380=CARTESIAN_POINT('Ctrl Pts',(3.5,30.7531999223435,0.0564772772052952));
#5381=CARTESIAN_POINT('Ctrl Pts',(3.4816494202464,30.8781999223435,1.19369621402047));
#5382=CARTESIAN_POINT('Ctrl Pts',(2.79836296968141,31.0031999223435,2.10293946007876));
#5383=CARTESIAN_POINT('Ctrl Pts',(2.11507651911643,31.1281999223435,3.01218270613706));
#5384=CARTESIAN_POINT('Ctrl Pts',(1.02784639780361,31.2531999223435,3.3461502454855));
#5385=CARTESIAN_POINT('Ctrl Pts',(-0.0593837235092006,31.3781999223435,
3.68011778483394));
#5386=CARTESIAN_POINT('Ctrl Pts',(-1.13527256282102,31.5031999223435,3.31124536858058));
#5387=CARTESIAN_POINT('Ctrl Pts',(-2.21116140213284,31.6281999223435,2.94237295232722));
#5388=CARTESIAN_POINT('Ctrl Pts',(-2.86475599094322,31.7531999223435,2.01155730596855));
#5389=CARTESIAN_POINT('Ctrl Pts',(-3.51835057975361,31.8781999223435,1.08074165960988));
#5390=CARTESIAN_POINT('Ctrl Pts',(-3.5,32.0031999223435,-0.0564772772052956));
#5391=CARTESIAN_POINT('Ctrl Pts',(-3.4816494202464,32.1281999223435,-1.19369621402047));
#5392=CARTESIAN_POINT('Ctrl Pts',(-2.79836296968141,32.2531999223435,-2.10293946007877));
#5393=CARTESIAN_POINT('Ctrl Pts',(-2.11507651911643,32.3781999223436,-3.01218270613706));
#5394=CARTESIAN_POINT('Ctrl Pts',(-1.02784639780361,32.5031999223435,-3.3461502454855));
#5395=CARTESIAN_POINT('Ctrl Pts',(0.0593837235092011,32.6281999223435,-3.68011778483394));
#5396=CARTESIAN_POINT('Ctrl Pts',(1.13527256282102,32.7531999223435,-3.31124536858058));
#5397=CARTESIAN_POINT('Ctrl Pts',(2.21116140213284,32.8781999223435,-2.94237295232722));
#5398=CARTESIAN_POINT('Ctrl Pts',(2.86475599094322,33.0031999223436,-2.01155730596855));
#5399=CARTESIAN_POINT('Ctrl Pts',(3.51835057975361,33.1281999223435,-1.08074165960988));
#5400=CARTESIAN_POINT('Ctrl Pts',(3.5,33.2531999223435,0.0564772772052952));
#5401=CARTESIAN_POINT('Ctrl Pts',(3.4816494202464,33.3781999223435,1.19369621402047));
#5402=CARTESIAN_POINT('Ctrl Pts',(2.79836296968141,33.5031999223435,2.10293946007876));
#5403=CARTESIAN_POINT('Ctrl Pts',(2.11507651911643,33.6281999223435,3.01218270613706));
#5404=CARTESIAN_POINT('Ctrl Pts',(1.02784639780361,33.7531999223435,3.3461502454855));
#5405=CARTESIAN_POINT('Ctrl Pts',(-0.0593837235092006,33.8781999223435,
3.68011778483394));
#5406=CARTESIAN_POINT('Ctrl Pts',(-1.13527256282102,34.0031999223435,3.31124536858058));
#5407=CARTESIAN_POINT('Ctrl Pts',(-2.21116140213284,34.1281999223435,2.94237295232722));
#5408=CARTESIAN_POINT('Ctrl Pts',(-2.86475599094322,34.2531999223436,2.01155730596855));
#5409=CARTESIAN_POINT('Ctrl Pts',(-3.51835057975361,34.3781999223435,1.08074165960988));
#5410=CARTESIAN_POINT('Ctrl Pts',(-3.5,34.5031999223435,-0.0564772772052956));
#5411=CARTESIAN_POINT('Ctrl Pts',(-3.4816494202464,34.6281999223435,-1.19369621402047));
#5412=CARTESIAN_POINT('Ctrl Pts',(-2.79836296968141,34.7531999223435,-2.10293946007877));
#5413=CARTESIAN_POINT('Ctrl Pts',(-2.11507651911643,34.8781999223436,-3.01218270613706));
#5414=CARTESIAN_POINT('Ctrl Pts',(-1.02784639780361,35.0031999223435,-3.3461502454855));
#5415=CARTESIAN_POINT('Ctrl Pts',(0.0593837235092011,35.1281999223435,-3.68011778483394));
#5416=CARTESIAN_POINT('Ctrl Pts',(1.13527256282102,35.2531999223435,-3.31124536858058));
#5417=CARTESIAN_POINT('Ctrl Pts',(2.21116140213284,35.3781999223435,-2.94237295232722));
#5418=CARTESIAN_POINT('Ctrl Pts',(2.86475599094322,35.5031999223436,-2.01155730596855));
#5419=CARTESIAN_POINT('Ctrl Pts',(3.51835057975361,35.6281999223435,-1.08074165960988));
#5420=CARTESIAN_POINT('Ctrl Pts',(3.5,35.7531999223435,0.0564772772052952));
#5421=CARTESIAN_POINT('Ctrl Pts',(3.4816494202464,35.8781999223435,1.19369621402047));
#5422=CARTESIAN_POINT('Ctrl Pts',(2.79836296968141,36.0031999223435,2.10293946007876));
#5423=CARTESIAN_POINT('Ctrl Pts',(2.11507651911643,36.1281999223436,3.01218270613706));
#5424=CARTESIAN_POINT('Ctrl Pts',(1.02784639780361,36.2531999223435,3.3461502454855));
#5425=CARTESIAN_POINT('Ctrl Pts',(-0.0593837235092006,36.3781999223435,
3.68011778483394));
#5426=CARTESIAN_POINT('Ctrl Pts',(-1.13527256282102,36.5031999223435,3.31124536858058));
#5427=CARTESIAN_POINT('Ctrl Pts',(-2.21116140213284,36.6281999223435,2.94237295232722));
#5428=CARTESIAN_POINT('Ctrl Pts',(-2.86475599094322,36.7531999223435,2.01155730596855));
#5429=CARTESIAN_POINT('Ctrl Pts',(-3.51835057975361,36.8781999223435,1.08074165960988));
#5430=CARTESIAN_POINT('Ctrl Pts',(-3.5,37.0031999223435,-0.0564772772052956));
#5431=CARTESIAN_POINT('Ctrl Pts',(-3.4816494202464,37.1281999223435,-1.19369621402047));
#5432=CARTESIAN_POINT('Ctrl Pts',(-2.79836296968141,37.2531999223435,-2.10293946007877));
#5433=CARTESIAN_POINT('Ctrl Pts',(-2.11507651911643,37.3781999223435,-3.01218270613706));
#5434=CARTESIAN_POINT('Ctrl Pts',(-1.02784639780361,37.5031999223435,-3.3461502454855));
#5435=CARTESIAN_POINT('Ctrl Pts',(0.0593837235092011,37.6281999223435,-3.68011778483394));
#5436=CARTESIAN_POINT('Ctrl Pts',(1.13527256282102,37.7531999223435,-3.31124536858058));
#5437=CARTESIAN_POINT('Ctrl Pts',(2.21116140213284,37.8781999223435,-2.94237295232722));
#5438=CARTESIAN_POINT('Ctrl Pts',(2.86475599094322,38.0031999223435,-2.01155730596855));
#5439=CARTESIAN_POINT('Ctrl Pts',(3.51835057975361,38.1281999223435,-1.08074165960988));
#5440=CARTESIAN_POINT('Ctrl Pts',(3.5,38.2531999223435,0.0564772772052952));
#5441=CARTESIAN_POINT('Ctrl Pts',(3.4816494202464,38.3781999223435,1.19369621402047));
#5442=CARTESIAN_POINT('Ctrl Pts',(2.79836296968141,38.5031999223435,2.10293946007876));
#5443=CARTESIAN_POINT('Ctrl Pts',(2.11507651911643,38.6281999223435,3.01218270613706));
#5444=CARTESIAN_POINT('Ctrl Pts',(1.02784639780361,38.7531999223435,3.3461502454855));
#5445=CARTESIAN_POINT('Ctrl Pts',(-0.0593837235092006,38.8781999223435,
3.68011778483394));
#5446=CARTESIAN_POINT('Ctrl Pts',(-1.13527256282102,39.0031999223435,3.31124536858058));
#5447=CARTESIAN_POINT('Ctrl Pts',(-2.21116140213284,39.1281999223435,2.94237295232722));
#5448=CARTESIAN_POINT('Ctrl Pts',(-2.86475599094322,39.2531999223436,2.01155730596855));
#5449=CARTESIAN_POINT('Ctrl Pts',(-3.51835057975361,39.3781999223435,1.08074165960988));
#5450=CARTESIAN_POINT('Ctrl Pts',(-3.5,39.5031999223435,-0.056477277205296));
#5451=CARTESIAN_POINT('',(-3.5,40.4968000776565,0.0564772772053685));
#5452=CARTESIAN_POINT('Origin',(-3.5,40.,3.664603343001E-14));
#5453=CARTESIAN_POINT('',(-3.5,15.4968000776565,0.056477277205369));
#5454=CARTESIAN_POINT('Ctrl Pts',(-3.5,15.4968000776565,0.056477277205369));
#5455=CARTESIAN_POINT('Ctrl Pts',(-3.51835057975363,15.6218000776565,-1.0807416596098));
#5456=CARTESIAN_POINT('Ctrl Pts',(-2.86475599094327,15.7468000776565,-2.01155730596849));
#5457=CARTESIAN_POINT('Ctrl Pts',(-2.2111614021329,15.8718000776565,-2.94237295232717));
#5458=CARTESIAN_POINT('Ctrl Pts',(-1.13527256282109,15.9968000776565,-3.31124536858055));
#5459=CARTESIAN_POINT('Ctrl Pts',(-0.0593837235092786,16.1218000776565,
-3.68011778483394));
#5460=CARTESIAN_POINT('Ctrl Pts',(1.02784639780354,16.2468000776565,-3.34615024548552));
#5461=CARTESIAN_POINT('Ctrl Pts',(2.11507651911636,16.3718000776565,-3.01218270613711));
#5462=CARTESIAN_POINT('Ctrl Pts',(2.79836296968137,16.4968000776565,-2.10293946007882));
#5463=CARTESIAN_POINT('Ctrl Pts',(3.48164942024637,16.6218000776565,-1.19369621402054));
#5464=CARTESIAN_POINT('Ctrl Pts',(3.5,16.7468000776565,-0.0564772772053694));
#5465=CARTESIAN_POINT('Ctrl Pts',(3.51835057975363,16.8718000776565,1.0807416596098));
#5466=CARTESIAN_POINT('Ctrl Pts',(2.86475599094327,16.9968000776565,2.01155730596849));
#5467=CARTESIAN_POINT('Ctrl Pts',(2.2111614021329,17.1218000776565,2.94237295232717));
#5468=CARTESIAN_POINT('Ctrl Pts',(1.13527256282109,17.2468000776565,3.31124536858055));
#5469=CARTESIAN_POINT('Ctrl Pts',(0.0593837235092791,17.3718000776565,3.68011778483394));
#5470=CARTESIAN_POINT('Ctrl Pts',(-1.02784639780354,17.4968000776565,3.34615024548552));
#5471=CARTESIAN_POINT('Ctrl Pts',(-2.11507651911636,17.6218000776565,3.01218270613711));
#5472=CARTESIAN_POINT('Ctrl Pts',(-2.79836296968137,17.7468000776565,2.10293946007882));
#5473=CARTESIAN_POINT('Ctrl Pts',(-3.48164942024637,17.8718000776565,1.19369621402054));
#5474=CARTESIAN_POINT('Ctrl Pts',(-3.5,17.9968000776565,0.0564772772053689));
#5475=CARTESIAN_POINT('Ctrl Pts',(-3.51835057975363,18.1218000776565,-1.0807416596098));
#5476=CARTESIAN_POINT('Ctrl Pts',(-2.86475599094327,18.2468000776565,-2.01155730596849));
#5477=CARTESIAN_POINT('Ctrl Pts',(-2.2111614021329,18.3718000776565,-2.94237295232717));
#5478=CARTESIAN_POINT('Ctrl Pts',(-1.13527256282109,18.4968000776565,-3.31124536858055));
#5479=CARTESIAN_POINT('Ctrl Pts',(-0.0593837235092786,18.6218000776565,
-3.68011778483394));
#5480=CARTESIAN_POINT('Ctrl Pts',(1.02784639780354,18.7468000776565,-3.34615024548552));
#5481=CARTESIAN_POINT('Ctrl Pts',(2.11507651911636,18.8718000776565,-3.01218270613711));
#5482=CARTESIAN_POINT('Ctrl Pts',(2.79836296968137,18.9968000776565,-2.10293946007882));
#5483=CARTESIAN_POINT('Ctrl Pts',(3.48164942024637,19.1218000776565,-1.19369621402054));
#5484=CARTESIAN_POINT('Ctrl Pts',(3.5,19.2468000776565,-0.0564772772053694));
#5485=CARTESIAN_POINT('Ctrl Pts',(3.51835057975363,19.3718000776565,1.0807416596098));
#5486=CARTESIAN_POINT('Ctrl Pts',(2.86475599094327,19.4968000776565,2.01155730596849));
#5487=CARTESIAN_POINT('Ctrl Pts',(2.2111614021329,19.6218000776565,2.94237295232717));
#5488=CARTESIAN_POINT('Ctrl Pts',(1.13527256282109,19.7468000776565,3.31124536858055));
#5489=CARTESIAN_POINT('Ctrl Pts',(0.0593837235092791,19.8718000776565,3.68011778483394));
#5490=CARTESIAN_POINT('Ctrl Pts',(-1.02784639780354,19.9968000776565,3.34615024548552));
#5491=CARTESIAN_POINT('Ctrl Pts',(-2.11507651911636,20.1218000776565,3.01218270613711));
#5492=CARTESIAN_POINT('Ctrl Pts',(-2.79836296968137,20.2468000776565,2.10293946007882));
#5493=CARTESIAN_POINT('Ctrl Pts',(-3.48164942024637,20.3718000776565,1.19369621402054));
#5494=CARTESIAN_POINT('Ctrl Pts',(-3.5,20.4968000776565,0.0564772772053689));
#5495=CARTESIAN_POINT('Ctrl Pts',(-3.51835057975363,20.6218000776565,-1.0807416596098));
#5496=CARTESIAN_POINT('Ctrl Pts',(-2.86475599094327,20.7468000776565,-2.01155730596849));
#5497=CARTESIAN_POINT('Ctrl Pts',(-2.2111614021329,20.8718000776565,-2.94237295232717));
#5498=CARTESIAN_POINT('Ctrl Pts',(-1.13527256282109,20.9968000776565,-3.31124536858055));
#5499=CARTESIAN_POINT('Ctrl Pts',(-0.0593837235092786,21.1218000776565,
-3.68011778483394));
#5500=CARTESIAN_POINT('Ctrl Pts',(1.02784639780354,21.2468000776565,-3.34615024548552));
#5501=CARTESIAN_POINT('Ctrl Pts',(2.11507651911636,21.3718000776565,-3.01218270613711));
#5502=CARTESIAN_POINT('Ctrl Pts',(2.79836296968137,21.4968000776565,-2.10293946007882));
#5503=CARTESIAN_POINT('Ctrl Pts',(3.48164942024637,21.6218000776565,-1.19369621402054));
#5504=CARTESIAN_POINT('Ctrl Pts',(3.5,21.7468000776565,-0.0564772772053694));
#5505=CARTESIAN_POINT('Ctrl Pts',(3.51835057975363,21.8718000776565,1.0807416596098));
#5506=CARTESIAN_POINT('Ctrl Pts',(2.86475599094327,21.9968000776565,2.01155730596849));
#5507=CARTESIAN_POINT('Ctrl Pts',(2.2111614021329,22.1218000776565,2.94237295232717));
#5508=CARTESIAN_POINT('Ctrl Pts',(1.13527256282109,22.2468000776565,3.31124536858055));
#5509=CARTESIAN_POINT('Ctrl Pts',(0.0593837235092791,22.3718000776565,3.68011778483394));
#5510=CARTESIAN_POINT('Ctrl Pts',(-1.02784639780354,22.4968000776565,3.34615024548552));
#5511=CARTESIAN_POINT('Ctrl Pts',(-2.11507651911636,22.6218000776565,3.01218270613711));
#5512=CARTESIAN_POINT('Ctrl Pts',(-2.79836296968137,22.7468000776565,2.10293946007882));
#5513=CARTESIAN_POINT('Ctrl Pts',(-3.48164942024637,22.8718000776565,1.19369621402054));
#5514=CARTESIAN_POINT('Ctrl Pts',(-3.5,22.9968000776565,0.0564772772053689));
#5515=CARTESIAN_POINT('Ctrl Pts',(-3.51835057975363,23.1218000776565,-1.0807416596098));
#5516=CARTESIAN_POINT('Ctrl Pts',(-2.86475599094327,23.2468000776565,-2.01155730596849));
#5517=CARTESIAN_POINT('Ctrl Pts',(-2.2111614021329,23.3718000776565,-2.94237295232717));
#5518=CARTESIAN_POINT('Ctrl Pts',(-1.13527256282109,23.4968000776565,-3.31124536858055));
#5519=CARTESIAN_POINT('Ctrl Pts',(-0.0593837235092786,23.6218000776565,
-3.68011778483394));
#5520=CARTESIAN_POINT('Ctrl Pts',(1.02784639780354,23.7468000776565,-3.34615024548552));
#5521=CARTESIAN_POINT('Ctrl Pts',(2.11507651911636,23.8718000776565,-3.01218270613711));
#5522=CARTESIAN_POINT('Ctrl Pts',(2.79836296968137,23.9968000776565,-2.10293946007882));
#5523=CARTESIAN_POINT('Ctrl Pts',(3.48164942024637,24.1218000776565,-1.19369621402054));
#5524=CARTESIAN_POINT('Ctrl Pts',(3.5,24.2468000776565,-0.0564772772053694));
#5525=CARTESIAN_POINT('Ctrl Pts',(3.51835057975363,24.3718000776565,1.0807416596098));
#5526=CARTESIAN_POINT('Ctrl Pts',(2.86475599094327,24.4968000776565,2.01155730596849));
#5527=CARTESIAN_POINT('Ctrl Pts',(2.2111614021329,24.6218000776565,2.94237295232717));
#5528=CARTESIAN_POINT('Ctrl Pts',(1.13527256282109,24.7468000776565,3.31124536858055));
#5529=CARTESIAN_POINT('Ctrl Pts',(0.0593837235092791,24.8718000776565,3.68011778483394));
#5530=CARTESIAN_POINT('Ctrl Pts',(-1.02784639780354,24.9968000776565,3.34615024548552));
#5531=CARTESIAN_POINT('Ctrl Pts',(-2.11507651911636,25.1218000776565,3.01218270613711));
#5532=CARTESIAN_POINT('Ctrl Pts',(-2.79836296968137,25.2468000776565,2.10293946007882));
#5533=CARTESIAN_POINT('Ctrl Pts',(-3.48164942024637,25.3718000776565,1.19369621402054));
#5534=CARTESIAN_POINT('Ctrl Pts',(-3.5,25.4968000776565,0.0564772772053689));
#5535=CARTESIAN_POINT('Ctrl Pts',(-3.51835057975363,25.6218000776565,-1.0807416596098));
#5536=CARTESIAN_POINT('Ctrl Pts',(-2.86475599094327,25.7468000776565,-2.01155730596849));
#5537=CARTESIAN_POINT('Ctrl Pts',(-2.2111614021329,25.8718000776565,-2.94237295232717));
#5538=CARTESIAN_POINT('Ctrl Pts',(-1.13527256282109,25.9968000776565,-3.31124536858055));
#5539=CARTESIAN_POINT('Ctrl Pts',(-0.0593837235092786,26.1218000776565,
-3.68011778483394));
#5540=CARTESIAN_POINT('Ctrl Pts',(1.02784639780354,26.2468000776565,-3.34615024548552));
#5541=CARTESIAN_POINT('Ctrl Pts',(2.11507651911636,26.3718000776565,-3.01218270613711));
#5542=CARTESIAN_POINT('Ctrl Pts',(2.79836296968137,26.4968000776565,-2.10293946007882));
#5543=CARTESIAN_POINT('Ctrl Pts',(3.48164942024637,26.6218000776565,-1.19369621402054));
#5544=CARTESIAN_POINT('Ctrl Pts',(3.5,26.7468000776565,-0.0564772772053694));
#5545=CARTESIAN_POINT('Ctrl Pts',(3.51835057975363,26.8718000776565,1.0807416596098));
#5546=CARTESIAN_POINT('Ctrl Pts',(2.86475599094327,26.9968000776565,2.01155730596849));
#5547=CARTESIAN_POINT('Ctrl Pts',(2.2111614021329,27.1218000776565,2.94237295232717));
#5548=CARTESIAN_POINT('Ctrl Pts',(1.13527256282109,27.2468000776565,3.31124536858055));
#5549=CARTESIAN_POINT('Ctrl Pts',(0.0593837235092791,27.3718000776565,3.68011778483394));
#5550=CARTESIAN_POINT('Ctrl Pts',(-1.02784639780354,27.4968000776565,3.34615024548552));
#5551=CARTESIAN_POINT('Ctrl Pts',(-2.11507651911636,27.6218000776565,3.01218270613711));
#5552=CARTESIAN_POINT('Ctrl Pts',(-2.79836296968137,27.7468000776565,2.10293946007882));
#5553=CARTESIAN_POINT('Ctrl Pts',(-3.48164942024637,27.8718000776565,1.19369621402054));
#5554=CARTESIAN_POINT('Ctrl Pts',(-3.5,27.9968000776565,0.0564772772053689));
#5555=CARTESIAN_POINT('Ctrl Pts',(-3.51835057975363,28.1218000776565,-1.0807416596098));
#5556=CARTESIAN_POINT('Ctrl Pts',(-2.86475599094327,28.2468000776565,-2.01155730596849));
#5557=CARTESIAN_POINT('Ctrl Pts',(-2.2111614021329,28.3718000776565,-2.94237295232717));
#5558=CARTESIAN_POINT('Ctrl Pts',(-1.13527256282109,28.4968000776565,-3.31124536858055));
#5559=CARTESIAN_POINT('Ctrl Pts',(-0.0593837235092786,28.6218000776565,
-3.68011778483394));
#5560=CARTESIAN_POINT('Ctrl Pts',(1.02784639780354,28.7468000776565,-3.34615024548552));
#5561=CARTESIAN_POINT('Ctrl Pts',(2.11507651911636,28.8718000776565,-3.01218270613711));
#5562=CARTESIAN_POINT('Ctrl Pts',(2.79836296968137,28.9968000776565,-2.10293946007882));
#5563=CARTESIAN_POINT('Ctrl Pts',(3.48164942024637,29.1218000776565,-1.19369621402054));
#5564=CARTESIAN_POINT('Ctrl Pts',(3.5,29.2468000776565,-0.0564772772053694));
#5565=CARTESIAN_POINT('Ctrl Pts',(3.51835057975363,29.3718000776565,1.0807416596098));
#5566=CARTESIAN_POINT('Ctrl Pts',(2.86475599094327,29.4968000776565,2.01155730596849));
#5567=CARTESIAN_POINT('Ctrl Pts',(2.2111614021329,29.6218000776565,2.94237295232717));
#5568=CARTESIAN_POINT('Ctrl Pts',(1.13527256282109,29.7468000776565,3.31124536858055));
#5569=CARTESIAN_POINT('Ctrl Pts',(0.0593837235092791,29.8718000776565,3.68011778483394));
#5570=CARTESIAN_POINT('Ctrl Pts',(-1.02784639780354,29.9968000776565,3.34615024548552));
#5571=CARTESIAN_POINT('Ctrl Pts',(-2.11507651911636,30.1218000776565,3.01218270613711));
#5572=CARTESIAN_POINT('Ctrl Pts',(-2.79836296968137,30.2468000776565,2.10293946007882));
#5573=CARTESIAN_POINT('Ctrl Pts',(-3.48164942024637,30.3718000776565,1.19369621402054));
#5574=CARTESIAN_POINT('Ctrl Pts',(-3.5,30.4968000776565,0.0564772772053689));
#5575=CARTESIAN_POINT('Ctrl Pts',(-3.51835057975363,30.6218000776565,-1.0807416596098));
#5576=CARTESIAN_POINT('Ctrl Pts',(-2.86475599094327,30.7468000776565,-2.01155730596849));
#5577=CARTESIAN_POINT('Ctrl Pts',(-2.2111614021329,30.8718000776565,-2.94237295232717));
#5578=CARTESIAN_POINT('Ctrl Pts',(-1.13527256282109,30.9968000776565,-3.31124536858055));
#5579=CARTESIAN_POINT('Ctrl Pts',(-0.0593837235092786,31.1218000776565,
-3.68011778483394));
#5580=CARTESIAN_POINT('Ctrl Pts',(1.02784639780354,31.2468000776565,-3.34615024548552));
#5581=CARTESIAN_POINT('Ctrl Pts',(2.11507651911636,31.3718000776565,-3.01218270613711));
#5582=CARTESIAN_POINT('Ctrl Pts',(2.79836296968137,31.4968000776565,-2.10293946007882));
#5583=CARTESIAN_POINT('Ctrl Pts',(3.48164942024637,31.6218000776565,-1.19369621402054));
#5584=CARTESIAN_POINT('Ctrl Pts',(3.5,31.7468000776565,-0.0564772772053694));
#5585=CARTESIAN_POINT('Ctrl Pts',(3.51835057975363,31.8718000776565,1.0807416596098));
#5586=CARTESIAN_POINT('Ctrl Pts',(2.86475599094327,31.9968000776565,2.01155730596849));
#5587=CARTESIAN_POINT('Ctrl Pts',(2.2111614021329,32.1218000776565,2.94237295232717));
#5588=CARTESIAN_POINT('Ctrl Pts',(1.13527256282109,32.2468000776565,3.31124536858055));
#5589=CARTESIAN_POINT('Ctrl Pts',(0.0593837235092791,32.3718000776565,3.68011778483394));
#5590=CARTESIAN_POINT('Ctrl Pts',(-1.02784639780354,32.4968000776565,3.34615024548552));
#5591=CARTESIAN_POINT('Ctrl Pts',(-2.11507651911636,32.6218000776565,3.01218270613711));
#5592=CARTESIAN_POINT('Ctrl Pts',(-2.79836296968137,32.7468000776565,2.10293946007882));
#5593=CARTESIAN_POINT('Ctrl Pts',(-3.48164942024637,32.8718000776565,1.19369621402054));
#5594=CARTESIAN_POINT('Ctrl Pts',(-3.5,32.9968000776565,0.0564772772053689));
#5595=CARTESIAN_POINT('Ctrl Pts',(-3.51835057975363,33.1218000776565,-1.0807416596098));
#5596=CARTESIAN_POINT('Ctrl Pts',(-2.86475599094327,33.2468000776565,-2.01155730596849));
#5597=CARTESIAN_POINT('Ctrl Pts',(-2.2111614021329,33.3718000776565,-2.94237295232717));
#5598=CARTESIAN_POINT('Ctrl Pts',(-1.13527256282109,33.4968000776565,-3.31124536858055));
#5599=CARTESIAN_POINT('Ctrl Pts',(-0.0593837235092786,33.6218000776565,
-3.68011778483394));
#5600=CARTESIAN_POINT('Ctrl Pts',(1.02784639780354,33.7468000776565,-3.34615024548552));
#5601=CARTESIAN_POINT('Ctrl Pts',(2.11507651911636,33.8718000776565,-3.01218270613711));
#5602=CARTESIAN_POINT('Ctrl Pts',(2.79836296968137,33.9968000776565,-2.10293946007882));
#5603=CARTESIAN_POINT('Ctrl Pts',(3.48164942024637,34.1218000776565,-1.19369621402054));
#5604=CARTESIAN_POINT('Ctrl Pts',(3.5,34.2468000776565,-0.0564772772053694));
#5605=CARTESIAN_POINT('Ctrl Pts',(3.51835057975363,34.3718000776565,1.0807416596098));
#5606=CARTESIAN_POINT('Ctrl Pts',(2.86475599094327,34.4968000776565,2.01155730596849));
#5607=CARTESIAN_POINT('Ctrl Pts',(2.2111614021329,34.6218000776565,2.94237295232717));
#5608=CARTESIAN_POINT('Ctrl Pts',(1.13527256282109,34.7468000776565,3.31124536858055));
#5609=CARTESIAN_POINT('Ctrl Pts',(0.0593837235092791,34.8718000776565,3.68011778483394));
#5610=CARTESIAN_POINT('Ctrl Pts',(-1.02784639780354,34.9968000776565,3.34615024548552));
#5611=CARTESIAN_POINT('Ctrl Pts',(-2.11507651911636,35.1218000776565,3.01218270613711));
#5612=CARTESIAN_POINT('Ctrl Pts',(-2.79836296968137,35.2468000776565,2.10293946007882));
#5613=CARTESIAN_POINT('Ctrl Pts',(-3.48164942024637,35.3718000776565,1.19369621402054));
#5614=CARTESIAN_POINT('Ctrl Pts',(-3.5,35.4968000776565,0.0564772772053689));
#5615=CARTESIAN_POINT('Ctrl Pts',(-3.51835057975363,35.6218000776565,-1.0807416596098));
#5616=CARTESIAN_POINT('Ctrl Pts',(-2.86475599094327,35.7468000776565,-2.01155730596849));
#5617=CARTESIAN_POINT('Ctrl Pts',(-2.2111614021329,35.8718000776565,-2.94237295232717));
#5618=CARTESIAN_POINT('Ctrl Pts',(-1.13527256282109,35.9968000776565,-3.31124536858055));
#5619=CARTESIAN_POINT('Ctrl Pts',(-0.0593837235092786,36.1218000776565,
-3.68011778483394));
#5620=CARTESIAN_POINT('Ctrl Pts',(1.02784639780354,36.2468000776565,-3.34615024548552));
#5621=CARTESIAN_POINT('Ctrl Pts',(2.11507651911636,36.3718000776565,-3.01218270613711));
#5622=CARTESIAN_POINT('Ctrl Pts',(2.79836296968137,36.4968000776565,-2.10293946007882));
#5623=CARTESIAN_POINT('Ctrl Pts',(3.48164942024637,36.6218000776565,-1.19369621402054));
#5624=CARTESIAN_POINT('Ctrl Pts',(3.5,36.7468000776565,-0.0564772772053694));
#5625=CARTESIAN_POINT('Ctrl Pts',(3.51835057975363,36.8718000776565,1.0807416596098));
#5626=CARTESIAN_POINT('Ctrl Pts',(2.86475599094327,36.9968000776565,2.01155730596849));
#5627=CARTESIAN_POINT('Ctrl Pts',(2.2111614021329,37.1218000776565,2.94237295232717));
#5628=CARTESIAN_POINT('Ctrl Pts',(1.13527256282109,37.2468000776565,3.31124536858055));
#5629=CARTESIAN_POINT('Ctrl Pts',(0.0593837235092791,37.3718000776565,3.68011778483394));
#5630=CARTESIAN_POINT('Ctrl Pts',(-1.02784639780354,37.4968000776565,3.34615024548552));
#5631=CARTESIAN_POINT('Ctrl Pts',(-2.11507651911636,37.6218000776565,3.01218270613711));
#5632=CARTESIAN_POINT('Ctrl Pts',(-2.79836296968137,37.7468000776565,2.10293946007882));
#5633=CARTESIAN_POINT('Ctrl Pts',(-3.48164942024637,37.8718000776565,1.19369621402054));
#5634=CARTESIAN_POINT('Ctrl Pts',(-3.5,37.9968000776565,0.0564772772053689));
#5635=CARTESIAN_POINT('Ctrl Pts',(-3.51835057975363,38.1218000776565,-1.0807416596098));
#5636=CARTESIAN_POINT('Ctrl Pts',(-2.86475599094327,38.2468000776565,-2.01155730596849));
#5637=CARTESIAN_POINT('Ctrl Pts',(-2.2111614021329,38.3718000776565,-2.94237295232717));
#5638=CARTESIAN_POINT('Ctrl Pts',(-1.13527256282109,38.4968000776565,-3.31124536858055));
#5639=CARTESIAN_POINT('Ctrl Pts',(-0.0593837235092786,38.6218000776565,
-3.68011778483394));
#5640=CARTESIAN_POINT('Ctrl Pts',(1.02784639780354,38.7468000776565,-3.34615024548552));
#5641=CARTESIAN_POINT('Ctrl Pts',(2.11507651911636,38.8718000776565,-3.01218270613711));
#5642=CARTESIAN_POINT('Ctrl Pts',(2.79836296968137,38.9968000776565,-2.10293946007882));
#5643=CARTESIAN_POINT('Ctrl Pts',(3.48164942024637,39.1218000776565,-1.19369621402054));
#5644=CARTESIAN_POINT('Ctrl Pts',(3.5,39.2468000776565,-0.0564772772053694));
#5645=CARTESIAN_POINT('Ctrl Pts',(3.51835057975363,39.3718000776565,1.0807416596098));
#5646=CARTESIAN_POINT('Ctrl Pts',(2.86475599094327,39.4968000776565,2.01155730596849));
#5647=CARTESIAN_POINT('Ctrl Pts',(2.2111614021329,39.6218000776565,2.94237295232717));
#5648=CARTESIAN_POINT('Ctrl Pts',(1.13527256282109,39.7468000776565,3.31124536858055));
#5649=CARTESIAN_POINT('Ctrl Pts',(0.0593837235092791,39.8718000776565,3.68011778483394));
#5650=CARTESIAN_POINT('Ctrl Pts',(-1.02784639780354,39.9968000776565,3.34615024548552));
#5651=CARTESIAN_POINT('Ctrl Pts',(-2.11507651911636,40.1218000776565,3.01218270613711));
#5652=CARTESIAN_POINT('Ctrl Pts',(-2.79836296968137,40.2468000776565,2.10293946007882));
#5653=CARTESIAN_POINT('Ctrl Pts',(-3.48164942024637,40.3718000776565,1.19369621402054));
#5654=CARTESIAN_POINT('Ctrl Pts',(-3.5,40.4968000776565,0.0564772772053685));
#5655=CARTESIAN_POINT('Origin',(-3.5,15.,3.664603343001E-14));
#5656=CARTESIAN_POINT('Origin',(-3.5,14.5031999223435,-0.0564772772052956));
#5657=CARTESIAN_POINT('',(-4.,15.,4.08336756143419E-14));
#5658=CARTESIAN_POINT('',(-3.5,15.,3.5649922684039E-14));
#5659=CARTESIAN_POINT('Origin',(-3.5,15.,3.664603343001E-14));
#5660=CARTESIAN_POINT('Origin',(-3.5,39.5031999223435,-0.0564772772052956));
#5661=CARTESIAN_POINT('Origin',(-3.5,40.,3.664603343001E-14));
#5662=CARTESIAN_POINT('Ctrl Pts',(-3.5,15.4968000776565,0.0564772772053689));
#5663=CARTESIAN_POINT('Ctrl Pts',(-3.51835057975363,15.6218000776565,-1.0807416596098));
#5664=CARTESIAN_POINT('Ctrl Pts',(-2.86475599094327,15.7468000776565,-2.01155730596849));
#5665=CARTESIAN_POINT('Ctrl Pts',(-2.2111614021329,15.8718000776565,-2.94237295232717));
#5666=CARTESIAN_POINT('Ctrl Pts',(-1.13527256282109,15.9968000776565,-3.31124536858055));
#5667=CARTESIAN_POINT('Ctrl Pts',(-0.0593837235092786,16.1218000776565,
-3.68011778483394));
#5668=CARTESIAN_POINT('Ctrl Pts',(1.02784639780354,16.2468000776565,-3.34615024548552));
#5669=CARTESIAN_POINT('Ctrl Pts',(2.11507651911636,16.3718000776565,-3.01218270613711));
#5670=CARTESIAN_POINT('Ctrl Pts',(2.79836296968137,16.4968000776565,-2.10293946007882));
#5671=CARTESIAN_POINT('Ctrl Pts',(3.48164942024637,16.6218000776565,-1.19369621402054));
#5672=CARTESIAN_POINT('Ctrl Pts',(3.5,16.7468000776565,-0.0564772772053694));
#5673=CARTESIAN_POINT('Ctrl Pts',(3.51835057975363,16.8718000776565,1.0807416596098));
#5674=CARTESIAN_POINT('Ctrl Pts',(2.86475599094327,16.9968000776565,2.01155730596849));
#5675=CARTESIAN_POINT('Ctrl Pts',(2.2111614021329,17.1218000776565,2.94237295232717));
#5676=CARTESIAN_POINT('Ctrl Pts',(1.13527256282109,17.2468000776565,3.31124536858055));
#5677=CARTESIAN_POINT('Ctrl Pts',(0.0593837235092791,17.3718000776565,3.68011778483394));
#5678=CARTESIAN_POINT('Ctrl Pts',(-1.02784639780354,17.4968000776565,3.34615024548552));
#5679=CARTESIAN_POINT('Ctrl Pts',(-2.11507651911636,17.6218000776565,3.01218270613711));
#5680=CARTESIAN_POINT('Ctrl Pts',(-2.79836296968137,17.7468000776565,2.10293946007882));
#5681=CARTESIAN_POINT('Ctrl Pts',(-3.48164942024637,17.8718000776565,1.19369621402054));
#5682=CARTESIAN_POINT('Ctrl Pts',(-3.5,17.9968000776565,0.0564772772053689));
#5683=CARTESIAN_POINT('Ctrl Pts',(-3.51835057975363,18.1218000776565,-1.0807416596098));
#5684=CARTESIAN_POINT('Ctrl Pts',(-2.86475599094327,18.2468000776565,-2.01155730596849));
#5685=CARTESIAN_POINT('Ctrl Pts',(-2.2111614021329,18.3718000776565,-2.94237295232717));
#5686=CARTESIAN_POINT('Ctrl Pts',(-1.13527256282109,18.4968000776565,-3.31124536858055));
#5687=CARTESIAN_POINT('Ctrl Pts',(-0.0593837235092786,18.6218000776565,
-3.68011778483394));
#5688=CARTESIAN_POINT('Ctrl Pts',(1.02784639780354,18.7468000776565,-3.34615024548552));
#5689=CARTESIAN_POINT('Ctrl Pts',(2.11507651911636,18.8718000776565,-3.01218270613711));
#5690=CARTESIAN_POINT('Ctrl Pts',(2.79836296968137,18.9968000776565,-2.10293946007882));
#5691=CARTESIAN_POINT('Ctrl Pts',(3.48164942024637,19.1218000776565,-1.19369621402054));
#5692=CARTESIAN_POINT('Ctrl Pts',(3.5,19.2468000776565,-0.0564772772053694));
#5693=CARTESIAN_POINT('Ctrl Pts',(3.51835057975363,19.3718000776565,1.0807416596098));
#5694=CARTESIAN_POINT('Ctrl Pts',(2.86475599094327,19.4968000776565,2.01155730596849));
#5695=CARTESIAN_POINT('Ctrl Pts',(2.2111614021329,19.6218000776565,2.94237295232717));
#5696=CARTESIAN_POINT('Ctrl Pts',(1.13527256282109,19.7468000776565,3.31124536858055));
#5697=CARTESIAN_POINT('Ctrl Pts',(0.0593837235092791,19.8718000776565,3.68011778483394));
#5698=CARTESIAN_POINT('Ctrl Pts',(-1.02784639780354,19.9968000776565,3.34615024548552));
#5699=CARTESIAN_POINT('Ctrl Pts',(-2.11507651911636,20.1218000776565,3.01218270613711));
#5700=CARTESIAN_POINT('Ctrl Pts',(-2.79836296968137,20.2468000776565,2.10293946007882));
#5701=CARTESIAN_POINT('Ctrl Pts',(-3.48164942024637,20.3718000776565,1.19369621402054));
#5702=CARTESIAN_POINT('Ctrl Pts',(-3.5,20.4968000776565,0.0564772772053689));
#5703=CARTESIAN_POINT('Ctrl Pts',(-3.51835057975363,20.6218000776565,-1.0807416596098));
#5704=CARTESIAN_POINT('Ctrl Pts',(-2.86475599094327,20.7468000776565,-2.01155730596849));
#5705=CARTESIAN_POINT('Ctrl Pts',(-2.2111614021329,20.8718000776565,-2.94237295232717));
#5706=CARTESIAN_POINT('Ctrl Pts',(-1.13527256282109,20.9968000776565,-3.31124536858055));
#5707=CARTESIAN_POINT('Ctrl Pts',(-0.0593837235092786,21.1218000776565,
-3.68011778483394));
#5708=CARTESIAN_POINT('Ctrl Pts',(1.02784639780354,21.2468000776565,-3.34615024548552));
#5709=CARTESIAN_POINT('Ctrl Pts',(2.11507651911636,21.3718000776565,-3.01218270613711));
#5710=CARTESIAN_POINT('Ctrl Pts',(2.79836296968137,21.4968000776565,-2.10293946007882));
#5711=CARTESIAN_POINT('Ctrl Pts',(3.48164942024637,21.6218000776565,-1.19369621402054));
#5712=CARTESIAN_POINT('Ctrl Pts',(3.5,21.7468000776565,-0.0564772772053694));
#5713=CARTESIAN_POINT('Ctrl Pts',(3.51835057975363,21.8718000776565,1.0807416596098));
#5714=CARTESIAN_POINT('Ctrl Pts',(2.86475599094327,21.9968000776565,2.01155730596849));
#5715=CARTESIAN_POINT('Ctrl Pts',(2.2111614021329,22.1218000776565,2.94237295232717));
#5716=CARTESIAN_POINT('Ctrl Pts',(1.13527256282109,22.2468000776565,3.31124536858055));
#5717=CARTESIAN_POINT('Ctrl Pts',(0.0593837235092791,22.3718000776565,3.68011778483394));
#5718=CARTESIAN_POINT('Ctrl Pts',(-1.02784639780354,22.4968000776565,3.34615024548552));
#5719=CARTESIAN_POINT('Ctrl Pts',(-2.11507651911636,22.6218000776565,3.01218270613711));
#5720=CARTESIAN_POINT('Ctrl Pts',(-2.79836296968137,22.7468000776565,2.10293946007882));
#5721=CARTESIAN_POINT('Ctrl Pts',(-3.48164942024637,22.8718000776565,1.19369621402054));
#5722=CARTESIAN_POINT('Ctrl Pts',(-3.5,22.9968000776565,0.0564772772053689));
#5723=CARTESIAN_POINT('Ctrl Pts',(-3.51835057975363,23.1218000776565,-1.0807416596098));
#5724=CARTESIAN_POINT('Ctrl Pts',(-2.86475599094327,23.2468000776565,-2.01155730596849));
#5725=CARTESIAN_POINT('Ctrl Pts',(-2.2111614021329,23.3718000776565,-2.94237295232717));
#5726=CARTESIAN_POINT('Ctrl Pts',(-1.13527256282109,23.4968000776565,-3.31124536858055));
#5727=CARTESIAN_POINT('Ctrl Pts',(-0.0593837235092786,23.6218000776565,
-3.68011778483394));
#5728=CARTESIAN_POINT('Ctrl Pts',(1.02784639780354,23.7468000776565,-3.34615024548552));
#5729=CARTESIAN_POINT('Ctrl Pts',(2.11507651911636,23.8718000776565,-3.01218270613711));
#5730=CARTESIAN_POINT('Ctrl Pts',(2.79836296968137,23.9968000776565,-2.10293946007882));
#5731=CARTESIAN_POINT('Ctrl Pts',(3.48164942024637,24.1218000776565,-1.19369621402054));
#5732=CARTESIAN_POINT('Ctrl Pts',(3.5,24.2468000776565,-0.0564772772053694));
#5733=CARTESIAN_POINT('Ctrl Pts',(3.51835057975363,24.3718000776565,1.0807416596098));
#5734=CARTESIAN_POINT('Ctrl Pts',(2.86475599094327,24.4968000776565,2.01155730596849));
#5735=CARTESIAN_POINT('Ctrl Pts',(2.2111614021329,24.6218000776565,2.94237295232717));
#5736=CARTESIAN_POINT('Ctrl Pts',(1.13527256282109,24.7468000776565,3.31124536858055));
#5737=CARTESIAN_POINT('Ctrl Pts',(0.0593837235092791,24.8718000776565,3.68011778483394));
#5738=CARTESIAN_POINT('Ctrl Pts',(-1.02784639780354,24.9968000776565,3.34615024548552));
#5739=CARTESIAN_POINT('Ctrl Pts',(-2.11507651911636,25.1218000776565,3.01218270613711));
#5740=CARTESIAN_POINT('Ctrl Pts',(-2.79836296968137,25.2468000776565,2.10293946007882));
#5741=CARTESIAN_POINT('Ctrl Pts',(-3.48164942024637,25.3718000776565,1.19369621402054));
#5742=CARTESIAN_POINT('Ctrl Pts',(-3.5,25.4968000776565,0.0564772772053689));
#5743=CARTESIAN_POINT('Ctrl Pts',(-3.51835057975363,25.6218000776565,-1.0807416596098));
#5744=CARTESIAN_POINT('Ctrl Pts',(-2.86475599094327,25.7468000776565,-2.01155730596849));
#5745=CARTESIAN_POINT('Ctrl Pts',(-2.2111614021329,25.8718000776565,-2.94237295232717));
#5746=CARTESIAN_POINT('Ctrl Pts',(-1.13527256282109,25.9968000776565,-3.31124536858055));
#5747=CARTESIAN_POINT('Ctrl Pts',(-0.0593837235092786,26.1218000776565,
-3.68011778483394));
#5748=CARTESIAN_POINT('Ctrl Pts',(1.02784639780354,26.2468000776565,-3.34615024548552));
#5749=CARTESIAN_POINT('Ctrl Pts',(2.11507651911636,26.3718000776565,-3.01218270613711));
#5750=CARTESIAN_POINT('Ctrl Pts',(2.79836296968137,26.4968000776565,-2.10293946007882));
#5751=CARTESIAN_POINT('Ctrl Pts',(3.48164942024637,26.6218000776565,-1.19369621402054));
#5752=CARTESIAN_POINT('Ctrl Pts',(3.5,26.7468000776565,-0.0564772772053694));
#5753=CARTESIAN_POINT('Ctrl Pts',(3.51835057975363,26.8718000776565,1.0807416596098));
#5754=CARTESIAN_POINT('Ctrl Pts',(2.86475599094327,26.9968000776565,2.01155730596849));
#5755=CARTESIAN_POINT('Ctrl Pts',(2.2111614021329,27.1218000776565,2.94237295232717));
#5756=CARTESIAN_POINT('Ctrl Pts',(1.13527256282109,27.2468000776565,3.31124536858055));
#5757=CARTESIAN_POINT('Ctrl Pts',(0.0593837235092791,27.3718000776565,3.68011778483394));
#5758=CARTESIAN_POINT('Ctrl Pts',(-1.02784639780354,27.4968000776565,3.34615024548552));
#5759=CARTESIAN_POINT('Ctrl Pts',(-2.11507651911636,27.6218000776565,3.01218270613711));
#5760=CARTESIAN_POINT('Ctrl Pts',(-2.79836296968137,27.7468000776565,2.10293946007882));
#5761=CARTESIAN_POINT('Ctrl Pts',(-3.48164942024637,27.8718000776565,1.19369621402054));
#5762=CARTESIAN_POINT('Ctrl Pts',(-3.5,27.9968000776565,0.0564772772053689));
#5763=CARTESIAN_POINT('Ctrl Pts',(-3.51835057975363,28.1218000776565,-1.0807416596098));
#5764=CARTESIAN_POINT('Ctrl Pts',(-2.86475599094327,28.2468000776565,-2.01155730596849));
#5765=CARTESIAN_POINT('Ctrl Pts',(-2.2111614021329,28.3718000776565,-2.94237295232717));
#5766=CARTESIAN_POINT('Ctrl Pts',(-1.13527256282109,28.4968000776565,-3.31124536858055));
#5767=CARTESIAN_POINT('Ctrl Pts',(-0.0593837235092786,28.6218000776565,
-3.68011778483394));
#5768=CARTESIAN_POINT('Ctrl Pts',(1.02784639780354,28.7468000776565,-3.34615024548552));
#5769=CARTESIAN_POINT('Ctrl Pts',(2.11507651911636,28.8718000776565,-3.01218270613711));
#5770=CARTESIAN_POINT('Ctrl Pts',(2.79836296968137,28.9968000776565,-2.10293946007882));
#5771=CARTESIAN_POINT('Ctrl Pts',(3.48164942024637,29.1218000776565,-1.19369621402054));
#5772=CARTESIAN_POINT('Ctrl Pts',(3.5,29.2468000776565,-0.0564772772053694));
#5773=CARTESIAN_POINT('Ctrl Pts',(3.51835057975363,29.3718000776565,1.0807416596098));
#5774=CARTESIAN_POINT('Ctrl Pts',(2.86475599094327,29.4968000776565,2.01155730596849));
#5775=CARTESIAN_POINT('Ctrl Pts',(2.2111614021329,29.6218000776565,2.94237295232717));
#5776=CARTESIAN_POINT('Ctrl Pts',(1.13527256282109,29.7468000776565,3.31124536858055));
#5777=CARTESIAN_POINT('Ctrl Pts',(0.0593837235092791,29.8718000776565,3.68011778483394));
#5778=CARTESIAN_POINT('Ctrl Pts',(-1.02784639780354,29.9968000776565,3.34615024548552));
#5779=CARTESIAN_POINT('Ctrl Pts',(-2.11507651911636,30.1218000776565,3.01218270613711));
#5780=CARTESIAN_POINT('Ctrl Pts',(-2.79836296968137,30.2468000776565,2.10293946007882));
#5781=CARTESIAN_POINT('Ctrl Pts',(-3.48164942024637,30.3718000776565,1.19369621402054));
#5782=CARTESIAN_POINT('Ctrl Pts',(-3.5,30.4968000776565,0.0564772772053689));
#5783=CARTESIAN_POINT('Ctrl Pts',(-3.51835057975363,30.6218000776565,-1.0807416596098));
#5784=CARTESIAN_POINT('Ctrl Pts',(-2.86475599094327,30.7468000776565,-2.01155730596849));
#5785=CARTESIAN_POINT('Ctrl Pts',(-2.2111614021329,30.8718000776565,-2.94237295232717));
#5786=CARTESIAN_POINT('Ctrl Pts',(-1.13527256282109,30.9968000776565,-3.31124536858055));
#5787=CARTESIAN_POINT('Ctrl Pts',(-0.0593837235092786,31.1218000776565,
-3.68011778483394));
#5788=CARTESIAN_POINT('Ctrl Pts',(1.02784639780354,31.2468000776565,-3.34615024548552));
#5789=CARTESIAN_POINT('Ctrl Pts',(2.11507651911636,31.3718000776565,-3.01218270613711));
#5790=CARTESIAN_POINT('Ctrl Pts',(2.79836296968137,31.4968000776565,-2.10293946007882));
#5791=CARTESIAN_POINT('Ctrl Pts',(3.48164942024637,31.6218000776565,-1.19369621402054));
#5792=CARTESIAN_POINT('Ctrl Pts',(3.5,31.7468000776565,-0.0564772772053694));
#5793=CARTESIAN_POINT('Ctrl Pts',(3.51835057975363,31.8718000776565,1.0807416596098));
#5794=CARTESIAN_POINT('Ctrl Pts',(2.86475599094327,31.9968000776565,2.01155730596849));
#5795=CARTESIAN_POINT('Ctrl Pts',(2.2111614021329,32.1218000776565,2.94237295232717));
#5796=CARTESIAN_POINT('Ctrl Pts',(1.13527256282109,32.2468000776565,3.31124536858055));
#5797=CARTESIAN_POINT('Ctrl Pts',(0.0593837235092791,32.3718000776565,3.68011778483394));
#5798=CARTESIAN_POINT('Ctrl Pts',(-1.02784639780354,32.4968000776565,3.34615024548552));
#5799=CARTESIAN_POINT('Ctrl Pts',(-2.11507651911636,32.6218000776565,3.01218270613711));
#5800=CARTESIAN_POINT('Ctrl Pts',(-2.79836296968137,32.7468000776565,2.10293946007882));
#5801=CARTESIAN_POINT('Ctrl Pts',(-3.48164942024637,32.8718000776565,1.19369621402054));
#5802=CARTESIAN_POINT('Ctrl Pts',(-3.5,32.9968000776565,0.0564772772053689));
#5803=CARTESIAN_POINT('Ctrl Pts',(-3.51835057975363,33.1218000776565,-1.0807416596098));
#5804=CARTESIAN_POINT('Ctrl Pts',(-2.86475599094327,33.2468000776565,-2.01155730596849));
#5805=CARTESIAN_POINT('Ctrl Pts',(-2.2111614021329,33.3718000776565,-2.94237295232717));
#5806=CARTESIAN_POINT('Ctrl Pts',(-1.13527256282109,33.4968000776565,-3.31124536858055));
#5807=CARTESIAN_POINT('Ctrl Pts',(-0.0593837235092786,33.6218000776565,
-3.68011778483394));
#5808=CARTESIAN_POINT('Ctrl Pts',(1.02784639780354,33.7468000776565,-3.34615024548552));
#5809=CARTESIAN_POINT('Ctrl Pts',(2.11507651911636,33.8718000776565,-3.01218270613711));
#5810=CARTESIAN_POINT('Ctrl Pts',(2.79836296968137,33.9968000776565,-2.10293946007882));
#5811=CARTESIAN_POINT('Ctrl Pts',(3.48164942024637,34.1218000776565,-1.19369621402054));
#5812=CARTESIAN_POINT('Ctrl Pts',(3.5,34.2468000776565,-0.0564772772053694));
#5813=CARTESIAN_POINT('Ctrl Pts',(3.51835057975363,34.3718000776565,1.0807416596098));
#5814=CARTESIAN_POINT('Ctrl Pts',(2.86475599094327,34.4968000776565,2.01155730596849));
#5815=CARTESIAN_POINT('Ctrl Pts',(2.2111614021329,34.6218000776565,2.94237295232717));
#5816=CARTESIAN_POINT('Ctrl Pts',(1.13527256282109,34.7468000776565,3.31124536858055));
#5817=CARTESIAN_POINT('Ctrl Pts',(0.0593837235092791,34.8718000776565,3.68011778483394));
#5818=CARTESIAN_POINT('Ctrl Pts',(-1.02784639780354,34.9968000776565,3.34615024548552));
#5819=CARTESIAN_POINT('Ctrl Pts',(-2.11507651911636,35.1218000776565,3.01218270613711));
#5820=CARTESIAN_POINT('Ctrl Pts',(-2.79836296968137,35.2468000776565,2.10293946007882));
#5821=CARTESIAN_POINT('Ctrl Pts',(-3.48164942024637,35.3718000776565,1.19369621402054));
#5822=CARTESIAN_POINT('Ctrl Pts',(-3.5,35.4968000776565,0.0564772772053689));
#5823=CARTESIAN_POINT('Ctrl Pts',(-3.51835057975363,35.6218000776565,-1.0807416596098));
#5824=CARTESIAN_POINT('Ctrl Pts',(-2.86475599094327,35.7468000776565,-2.01155730596849));
#5825=CARTESIAN_POINT('Ctrl Pts',(-2.2111614021329,35.8718000776565,-2.94237295232717));
#5826=CARTESIAN_POINT('Ctrl Pts',(-1.13527256282109,35.9968000776565,-3.31124536858055));
#5827=CARTESIAN_POINT('Ctrl Pts',(-0.0593837235092786,36.1218000776565,
-3.68011778483394));
#5828=CARTESIAN_POINT('Ctrl Pts',(1.02784639780354,36.2468000776565,-3.34615024548552));
#5829=CARTESIAN_POINT('Ctrl Pts',(2.11507651911636,36.3718000776565,-3.01218270613711));
#5830=CARTESIAN_POINT('Ctrl Pts',(2.79836296968137,36.4968000776565,-2.10293946007882));
#5831=CARTESIAN_POINT('Ctrl Pts',(3.48164942024637,36.6218000776565,-1.19369621402054));
#5832=CARTESIAN_POINT('Ctrl Pts',(3.5,36.7468000776565,-0.0564772772053694));
#5833=CARTESIAN_POINT('Ctrl Pts',(3.51835057975363,36.8718000776565,1.0807416596098));
#5834=CARTESIAN_POINT('Ctrl Pts',(2.86475599094327,36.9968000776565,2.01155730596849));
#5835=CARTESIAN_POINT('Ctrl Pts',(2.2111614021329,37.1218000776565,2.94237295232717));
#5836=CARTESIAN_POINT('Ctrl Pts',(1.13527256282109,37.2468000776565,3.31124536858055));
#5837=CARTESIAN_POINT('Ctrl Pts',(0.0593837235092791,37.3718000776565,3.68011778483394));
#5838=CARTESIAN_POINT('Ctrl Pts',(-1.02784639780354,37.4968000776565,3.34615024548552));
#5839=CARTESIAN_POINT('Ctrl Pts',(-2.11507651911636,37.6218000776565,3.01218270613711));
#5840=CARTESIAN_POINT('Ctrl Pts',(-2.79836296968137,37.7468000776565,2.10293946007882));
#5841=CARTESIAN_POINT('Ctrl Pts',(-3.48164942024637,37.8718000776565,1.19369621402054));
#5842=CARTESIAN_POINT('Ctrl Pts',(-3.5,37.9968000776565,0.0564772772053689));
#5843=CARTESIAN_POINT('Ctrl Pts',(-3.51835057975363,38.1218000776565,-1.0807416596098));
#5844=CARTESIAN_POINT('Ctrl Pts',(-2.86475599094327,38.2468000776565,-2.01155730596849));
#5845=CARTESIAN_POINT('Ctrl Pts',(-2.2111614021329,38.3718000776565,-2.94237295232717));
#5846=CARTESIAN_POINT('Ctrl Pts',(-1.13527256282109,38.4968000776565,-3.31124536858055));
#5847=CARTESIAN_POINT('Ctrl Pts',(-0.0593837235092786,38.6218000776565,
-3.68011778483394));
#5848=CARTESIAN_POINT('Ctrl Pts',(1.02784639780354,38.7468000776565,-3.34615024548552));
#5849=CARTESIAN_POINT('Ctrl Pts',(2.11507651911636,38.8718000776565,-3.01218270613711));
#5850=CARTESIAN_POINT('Ctrl Pts',(2.79836296968137,38.9968000776565,-2.10293946007882));
#5851=CARTESIAN_POINT('Ctrl Pts',(3.48164942024637,39.1218000776565,-1.19369621402054));
#5852=CARTESIAN_POINT('Ctrl Pts',(3.5,39.2468000776565,-0.0564772772053694));
#5853=CARTESIAN_POINT('Ctrl Pts',(3.51835057975363,39.3718000776565,1.0807416596098));
#5854=CARTESIAN_POINT('Ctrl Pts',(2.86475599094327,39.4968000776565,2.01155730596849));
#5855=CARTESIAN_POINT('Ctrl Pts',(2.2111614021329,39.6218000776565,2.94237295232717));
#5856=CARTESIAN_POINT('Ctrl Pts',(1.13527256282109,39.7468000776565,3.31124536858055));
#5857=CARTESIAN_POINT('Ctrl Pts',(0.0593837235092791,39.8718000776565,3.68011778483394));
#5858=CARTESIAN_POINT('Ctrl Pts',(-1.02784639780354,39.9968000776565,3.34615024548552));
#5859=CARTESIAN_POINT('Ctrl Pts',(-2.11507651911636,40.1218000776565,3.01218270613711));
#5860=CARTESIAN_POINT('Ctrl Pts',(-2.79836296968137,40.2468000776565,2.10293946007882));
#5861=CARTESIAN_POINT('Ctrl Pts',(-3.48164942024637,40.3718000776565,1.19369621402054));
#5862=CARTESIAN_POINT('Ctrl Pts',(-3.5,40.4968000776565,0.0564772772053689));
#5863=CARTESIAN_POINT('Ctrl Pts',(-2.5,15.4968000776565,0.0564772772053586));
#5864=CARTESIAN_POINT('Ctrl Pts',(-2.51835057975363,15.6218000776565,-0.755821963376908));
#5865=CARTESIAN_POINT('Ctrl Pts',(-2.05573899656831,15.7468000776565,-1.42377205367602));
#5866=CARTESIAN_POINT('Ctrl Pts',(-1.593127413383,15.8718000776565,-2.09172214397514));
#5867=CARTESIAN_POINT('Ctrl Pts',(-0.826255568446133,15.9968000776565,-2.3601888522854));
#5868=CARTESIAN_POINT('Ctrl Pts',(-0.0593837235092677,16.1218000776565,
-2.62865556059567));
#5869=CARTESIAN_POINT('Ctrl Pts',(0.718829403428605,16.2468000776565,-2.39509372919037));
#5870=CARTESIAN_POINT('Ctrl Pts',(1.49704253036648,16.3718000776565,-2.16153189778506));
#5871=CARTESIAN_POINT('Ctrl Pts',(1.98934597530643,16.4968000776565,-1.51515420778634));
#5872=CARTESIAN_POINT('Ctrl Pts',(2.48164942024637,16.6218000776565,-0.868776517787625));
#5873=CARTESIAN_POINT('Ctrl Pts',(2.5,16.7468000776565,-0.0564772772053589));
#5874=CARTESIAN_POINT('Ctrl Pts',(2.51835057975363,16.8718000776565,0.755821963376907));
#5875=CARTESIAN_POINT('Ctrl Pts',(2.05573899656831,16.9968000776565,1.42377205367602));
#5876=CARTESIAN_POINT('Ctrl Pts',(1.593127413383,17.1218000776565,2.09172214397514));
#5877=CARTESIAN_POINT('Ctrl Pts',(0.826255568446133,17.2468000776565,2.3601888522854));
#5878=CARTESIAN_POINT('Ctrl Pts',(0.059383723509268,17.3718000776565,2.62865556059567));
#5879=CARTESIAN_POINT('Ctrl Pts',(-0.718829403428604,17.4968000776565,2.39509372919037));
#5880=CARTESIAN_POINT('Ctrl Pts',(-1.49704253036648,17.6218000776565,2.16153189778506));
#5881=CARTESIAN_POINT('Ctrl Pts',(-1.98934597530643,17.7468000776565,1.51515420778634));
#5882=CARTESIAN_POINT('Ctrl Pts',(-2.48164942024637,17.8718000776565,0.868776517787626));
#5883=CARTESIAN_POINT('Ctrl Pts',(-2.5,17.9968000776565,0.0564772772053586));
#5884=CARTESIAN_POINT('Ctrl Pts',(-2.51835057975363,18.1218000776565,-0.755821963376908));
#5885=CARTESIAN_POINT('Ctrl Pts',(-2.05573899656831,18.2468000776565,-1.42377205367602));
#5886=CARTESIAN_POINT('Ctrl Pts',(-1.593127413383,18.3718000776565,-2.09172214397514));
#5887=CARTESIAN_POINT('Ctrl Pts',(-0.826255568446133,18.4968000776565,-2.3601888522854));
#5888=CARTESIAN_POINT('Ctrl Pts',(-0.0593837235092677,18.6218000776565,
-2.62865556059567));
#5889=CARTESIAN_POINT('Ctrl Pts',(0.718829403428605,18.7468000776565,-2.39509372919037));
#5890=CARTESIAN_POINT('Ctrl Pts',(1.49704253036648,18.8718000776565,-2.16153189778506));
#5891=CARTESIAN_POINT('Ctrl Pts',(1.98934597530643,18.9968000776565,-1.51515420778634));
#5892=CARTESIAN_POINT('Ctrl Pts',(2.48164942024637,19.1218000776565,-0.868776517787625));
#5893=CARTESIAN_POINT('Ctrl Pts',(2.5,19.2468000776565,-0.0564772772053589));
#5894=CARTESIAN_POINT('Ctrl Pts',(2.51835057975363,19.3718000776565,0.755821963376907));
#5895=CARTESIAN_POINT('Ctrl Pts',(2.05573899656831,19.4968000776565,1.42377205367602));
#5896=CARTESIAN_POINT('Ctrl Pts',(1.593127413383,19.6218000776565,2.09172214397514));
#5897=CARTESIAN_POINT('Ctrl Pts',(0.826255568446133,19.7468000776565,2.3601888522854));
#5898=CARTESIAN_POINT('Ctrl Pts',(0.059383723509268,19.8718000776565,2.62865556059567));
#5899=CARTESIAN_POINT('Ctrl Pts',(-0.718829403428604,19.9968000776565,2.39509372919037));
#5900=CARTESIAN_POINT('Ctrl Pts',(-1.49704253036648,20.1218000776565,2.16153189778506));
#5901=CARTESIAN_POINT('Ctrl Pts',(-1.98934597530643,20.2468000776565,1.51515420778634));
#5902=CARTESIAN_POINT('Ctrl Pts',(-2.48164942024637,20.3718000776565,0.868776517787626));
#5903=CARTESIAN_POINT('Ctrl Pts',(-2.5,20.4968000776565,0.0564772772053586));
#5904=CARTESIAN_POINT('Ctrl Pts',(-2.51835057975363,20.6218000776565,-0.755821963376908));
#5905=CARTESIAN_POINT('Ctrl Pts',(-2.05573899656831,20.7468000776565,-1.42377205367602));
#5906=CARTESIAN_POINT('Ctrl Pts',(-1.593127413383,20.8718000776565,-2.09172214397514));
#5907=CARTESIAN_POINT('Ctrl Pts',(-0.826255568446133,20.9968000776565,-2.3601888522854));
#5908=CARTESIAN_POINT('Ctrl Pts',(-0.0593837235092677,21.1218000776565,
-2.62865556059567));
#5909=CARTESIAN_POINT('Ctrl Pts',(0.718829403428605,21.2468000776565,-2.39509372919037));
#5910=CARTESIAN_POINT('Ctrl Pts',(1.49704253036648,21.3718000776565,-2.16153189778506));
#5911=CARTESIAN_POINT('Ctrl Pts',(1.98934597530643,21.4968000776565,-1.51515420778634));
#5912=CARTESIAN_POINT('Ctrl Pts',(2.48164942024637,21.6218000776565,-0.868776517787625));
#5913=CARTESIAN_POINT('Ctrl Pts',(2.5,21.7468000776565,-0.0564772772053589));
#5914=CARTESIAN_POINT('Ctrl Pts',(2.51835057975363,21.8718000776565,0.755821963376907));
#5915=CARTESIAN_POINT('Ctrl Pts',(2.05573899656831,21.9968000776565,1.42377205367602));
#5916=CARTESIAN_POINT('Ctrl Pts',(1.593127413383,22.1218000776565,2.09172214397514));
#5917=CARTESIAN_POINT('Ctrl Pts',(0.826255568446133,22.2468000776565,2.3601888522854));
#5918=CARTESIAN_POINT('Ctrl Pts',(0.059383723509268,22.3718000776565,2.62865556059567));
#5919=CARTESIAN_POINT('Ctrl Pts',(-0.718829403428604,22.4968000776565,2.39509372919037));
#5920=CARTESIAN_POINT('Ctrl Pts',(-1.49704253036648,22.6218000776565,2.16153189778506));
#5921=CARTESIAN_POINT('Ctrl Pts',(-1.98934597530643,22.7468000776565,1.51515420778634));
#5922=CARTESIAN_POINT('Ctrl Pts',(-2.48164942024637,22.8718000776565,0.868776517787626));
#5923=CARTESIAN_POINT('Ctrl Pts',(-2.5,22.9968000776565,0.0564772772053586));
#5924=CARTESIAN_POINT('Ctrl Pts',(-2.51835057975363,23.1218000776565,-0.755821963376908));
#5925=CARTESIAN_POINT('Ctrl Pts',(-2.05573899656831,23.2468000776565,-1.42377205367602));
#5926=CARTESIAN_POINT('Ctrl Pts',(-1.593127413383,23.3718000776565,-2.09172214397514));
#5927=CARTESIAN_POINT('Ctrl Pts',(-0.826255568446133,23.4968000776565,-2.3601888522854));
#5928=CARTESIAN_POINT('Ctrl Pts',(-0.0593837235092677,23.6218000776565,
-2.62865556059567));
#5929=CARTESIAN_POINT('Ctrl Pts',(0.718829403428605,23.7468000776565,-2.39509372919037));
#5930=CARTESIAN_POINT('Ctrl Pts',(1.49704253036648,23.8718000776565,-2.16153189778506));
#5931=CARTESIAN_POINT('Ctrl Pts',(1.98934597530643,23.9968000776565,-1.51515420778634));
#5932=CARTESIAN_POINT('Ctrl Pts',(2.48164942024637,24.1218000776565,-0.868776517787625));
#5933=CARTESIAN_POINT('Ctrl Pts',(2.5,24.2468000776565,-0.0564772772053589));
#5934=CARTESIAN_POINT('Ctrl Pts',(2.51835057975363,24.3718000776565,0.755821963376907));
#5935=CARTESIAN_POINT('Ctrl Pts',(2.05573899656831,24.4968000776565,1.42377205367602));
#5936=CARTESIAN_POINT('Ctrl Pts',(1.593127413383,24.6218000776565,2.09172214397514));
#5937=CARTESIAN_POINT('Ctrl Pts',(0.826255568446133,24.7468000776565,2.3601888522854));
#5938=CARTESIAN_POINT('Ctrl Pts',(0.059383723509268,24.8718000776565,2.62865556059567));
#5939=CARTESIAN_POINT('Ctrl Pts',(-0.718829403428604,24.9968000776565,2.39509372919037));
#5940=CARTESIAN_POINT('Ctrl Pts',(-1.49704253036648,25.1218000776565,2.16153189778506));
#5941=CARTESIAN_POINT('Ctrl Pts',(-1.98934597530643,25.2468000776565,1.51515420778634));
#5942=CARTESIAN_POINT('Ctrl Pts',(-2.48164942024637,25.3718000776565,0.868776517787626));
#5943=CARTESIAN_POINT('Ctrl Pts',(-2.5,25.4968000776565,0.0564772772053586));
#5944=CARTESIAN_POINT('Ctrl Pts',(-2.51835057975363,25.6218000776565,-0.755821963376908));
#5945=CARTESIAN_POINT('Ctrl Pts',(-2.05573899656831,25.7468000776565,-1.42377205367602));
#5946=CARTESIAN_POINT('Ctrl Pts',(-1.593127413383,25.8718000776565,-2.09172214397514));
#5947=CARTESIAN_POINT('Ctrl Pts',(-0.826255568446133,25.9968000776565,-2.3601888522854));
#5948=CARTESIAN_POINT('Ctrl Pts',(-0.0593837235092677,26.1218000776565,
-2.62865556059567));
#5949=CARTESIAN_POINT('Ctrl Pts',(0.718829403428605,26.2468000776565,-2.39509372919037));
#5950=CARTESIAN_POINT('Ctrl Pts',(1.49704253036648,26.3718000776565,-2.16153189778506));
#5951=CARTESIAN_POINT('Ctrl Pts',(1.98934597530643,26.4968000776565,-1.51515420778634));
#5952=CARTESIAN_POINT('Ctrl Pts',(2.48164942024637,26.6218000776565,-0.868776517787625));
#5953=CARTESIAN_POINT('Ctrl Pts',(2.5,26.7468000776565,-0.0564772772053589));
#5954=CARTESIAN_POINT('Ctrl Pts',(2.51835057975363,26.8718000776565,0.755821963376907));
#5955=CARTESIAN_POINT('Ctrl Pts',(2.05573899656831,26.9968000776565,1.42377205367602));
#5956=CARTESIAN_POINT('Ctrl Pts',(1.593127413383,27.1218000776565,2.09172214397514));
#5957=CARTESIAN_POINT('Ctrl Pts',(0.826255568446133,27.2468000776565,2.3601888522854));
#5958=CARTESIAN_POINT('Ctrl Pts',(0.059383723509268,27.3718000776565,2.62865556059567));
#5959=CARTESIAN_POINT('Ctrl Pts',(-0.718829403428604,27.4968000776565,2.39509372919037));
#5960=CARTESIAN_POINT('Ctrl Pts',(-1.49704253036648,27.6218000776565,2.16153189778506));
#5961=CARTESIAN_POINT('Ctrl Pts',(-1.98934597530643,27.7468000776565,1.51515420778634));
#5962=CARTESIAN_POINT('Ctrl Pts',(-2.48164942024637,27.8718000776565,0.868776517787626));
#5963=CARTESIAN_POINT('Ctrl Pts',(-2.5,27.9968000776565,0.0564772772053586));
#5964=CARTESIAN_POINT('Ctrl Pts',(-2.51835057975363,28.1218000776565,-0.755821963376908));
#5965=CARTESIAN_POINT('Ctrl Pts',(-2.05573899656831,28.2468000776565,-1.42377205367602));
#5966=CARTESIAN_POINT('Ctrl Pts',(-1.593127413383,28.3718000776565,-2.09172214397514));
#5967=CARTESIAN_POINT('Ctrl Pts',(-0.826255568446133,28.4968000776565,-2.3601888522854));
#5968=CARTESIAN_POINT('Ctrl Pts',(-0.0593837235092677,28.6218000776565,
-2.62865556059567));
#5969=CARTESIAN_POINT('Ctrl Pts',(0.718829403428605,28.7468000776565,-2.39509372919037));
#5970=CARTESIAN_POINT('Ctrl Pts',(1.49704253036648,28.8718000776565,-2.16153189778506));
#5971=CARTESIAN_POINT('Ctrl Pts',(1.98934597530643,28.9968000776565,-1.51515420778634));
#5972=CARTESIAN_POINT('Ctrl Pts',(2.48164942024637,29.1218000776565,-0.868776517787625));
#5973=CARTESIAN_POINT('Ctrl Pts',(2.5,29.2468000776565,-0.0564772772053589));
#5974=CARTESIAN_POINT('Ctrl Pts',(2.51835057975363,29.3718000776565,0.755821963376907));
#5975=CARTESIAN_POINT('Ctrl Pts',(2.05573899656831,29.4968000776565,1.42377205367602));
#5976=CARTESIAN_POINT('Ctrl Pts',(1.593127413383,29.6218000776565,2.09172214397514));
#5977=CARTESIAN_POINT('Ctrl Pts',(0.826255568446133,29.7468000776565,2.3601888522854));
#5978=CARTESIAN_POINT('Ctrl Pts',(0.059383723509268,29.8718000776565,2.62865556059567));
#5979=CARTESIAN_POINT('Ctrl Pts',(-0.718829403428604,29.9968000776565,2.39509372919037));
#5980=CARTESIAN_POINT('Ctrl Pts',(-1.49704253036648,30.1218000776565,2.16153189778506));
#5981=CARTESIAN_POINT('Ctrl Pts',(-1.98934597530643,30.2468000776565,1.51515420778634));
#5982=CARTESIAN_POINT('Ctrl Pts',(-2.48164942024637,30.3718000776565,0.868776517787626));
#5983=CARTESIAN_POINT('Ctrl Pts',(-2.5,30.4968000776565,0.0564772772053586));
#5984=CARTESIAN_POINT('Ctrl Pts',(-2.51835057975363,30.6218000776565,-0.755821963376908));
#5985=CARTESIAN_POINT('Ctrl Pts',(-2.05573899656831,30.7468000776565,-1.42377205367602));
#5986=CARTESIAN_POINT('Ctrl Pts',(-1.593127413383,30.8718000776565,-2.09172214397514));
#5987=CARTESIAN_POINT('Ctrl Pts',(-0.826255568446133,30.9968000776565,-2.3601888522854));
#5988=CARTESIAN_POINT('Ctrl Pts',(-0.0593837235092677,31.1218000776565,
-2.62865556059567));
#5989=CARTESIAN_POINT('Ctrl Pts',(0.718829403428605,31.2468000776565,-2.39509372919037));
#5990=CARTESIAN_POINT('Ctrl Pts',(1.49704253036648,31.3718000776565,-2.16153189778506));
#5991=CARTESIAN_POINT('Ctrl Pts',(1.98934597530643,31.4968000776565,-1.51515420778634));
#5992=CARTESIAN_POINT('Ctrl Pts',(2.48164942024637,31.6218000776565,-0.868776517787625));
#5993=CARTESIAN_POINT('Ctrl Pts',(2.5,31.7468000776565,-0.0564772772053589));
#5994=CARTESIAN_POINT('Ctrl Pts',(2.51835057975363,31.8718000776565,0.755821963376907));
#5995=CARTESIAN_POINT('Ctrl Pts',(2.05573899656831,31.9968000776565,1.42377205367602));
#5996=CARTESIAN_POINT('Ctrl Pts',(1.593127413383,32.1218000776565,2.09172214397514));
#5997=CARTESIAN_POINT('Ctrl Pts',(0.826255568446133,32.2468000776565,2.3601888522854));
#5998=CARTESIAN_POINT('Ctrl Pts',(0.059383723509268,32.3718000776565,2.62865556059567));
#5999=CARTESIAN_POINT('Ctrl Pts',(-0.718829403428604,32.4968000776565,2.39509372919037));
#6000=CARTESIAN_POINT('Ctrl Pts',(-1.49704253036648,32.6218000776565,2.16153189778506));
#6001=CARTESIAN_POINT('Ctrl Pts',(-1.98934597530643,32.7468000776565,1.51515420778634));
#6002=CARTESIAN_POINT('Ctrl Pts',(-2.48164942024637,32.8718000776565,0.868776517787626));
#6003=CARTESIAN_POINT('Ctrl Pts',(-2.5,32.9968000776565,0.0564772772053586));
#6004=CARTESIAN_POINT('Ctrl Pts',(-2.51835057975363,33.1218000776565,-0.755821963376908));
#6005=CARTESIAN_POINT('Ctrl Pts',(-2.05573899656831,33.2468000776565,-1.42377205367602));
#6006=CARTESIAN_POINT('Ctrl Pts',(-1.593127413383,33.3718000776565,-2.09172214397514));
#6007=CARTESIAN_POINT('Ctrl Pts',(-0.826255568446133,33.4968000776565,-2.3601888522854));
#6008=CARTESIAN_POINT('Ctrl Pts',(-0.0593837235092677,33.6218000776565,
-2.62865556059567));
#6009=CARTESIAN_POINT('Ctrl Pts',(0.718829403428605,33.7468000776565,-2.39509372919037));
#6010=CARTESIAN_POINT('Ctrl Pts',(1.49704253036648,33.8718000776565,-2.16153189778506));
#6011=CARTESIAN_POINT('Ctrl Pts',(1.98934597530643,33.9968000776565,-1.51515420778634));
#6012=CARTESIAN_POINT('Ctrl Pts',(2.48164942024637,34.1218000776565,-0.868776517787625));
#6013=CARTESIAN_POINT('Ctrl Pts',(2.5,34.2468000776565,-0.0564772772053589));
#6014=CARTESIAN_POINT('Ctrl Pts',(2.51835057975363,34.3718000776565,0.755821963376907));
#6015=CARTESIAN_POINT('Ctrl Pts',(2.05573899656831,34.4968000776565,1.42377205367602));
#6016=CARTESIAN_POINT('Ctrl Pts',(1.593127413383,34.6218000776565,2.09172214397514));
#6017=CARTESIAN_POINT('Ctrl Pts',(0.826255568446133,34.7468000776565,2.3601888522854));
#6018=CARTESIAN_POINT('Ctrl Pts',(0.059383723509268,34.8718000776565,2.62865556059567));
#6019=CARTESIAN_POINT('Ctrl Pts',(-0.718829403428604,34.9968000776565,2.39509372919037));
#6020=CARTESIAN_POINT('Ctrl Pts',(-1.49704253036648,35.1218000776565,2.16153189778506));
#6021=CARTESIAN_POINT('Ctrl Pts',(-1.98934597530643,35.2468000776565,1.51515420778634));
#6022=CARTESIAN_POINT('Ctrl Pts',(-2.48164942024637,35.3718000776565,0.868776517787626));
#6023=CARTESIAN_POINT('Ctrl Pts',(-2.5,35.4968000776565,0.0564772772053586));
#6024=CARTESIAN_POINT('Ctrl Pts',(-2.51835057975363,35.6218000776565,-0.755821963376908));
#6025=CARTESIAN_POINT('Ctrl Pts',(-2.05573899656831,35.7468000776565,-1.42377205367602));
#6026=CARTESIAN_POINT('Ctrl Pts',(-1.593127413383,35.8718000776565,-2.09172214397514));
#6027=CARTESIAN_POINT('Ctrl Pts',(-0.826255568446133,35.9968000776565,-2.3601888522854));
#6028=CARTESIAN_POINT('Ctrl Pts',(-0.0593837235092677,36.1218000776565,
-2.62865556059567));
#6029=CARTESIAN_POINT('Ctrl Pts',(0.718829403428605,36.2468000776565,-2.39509372919037));
#6030=CARTESIAN_POINT('Ctrl Pts',(1.49704253036648,36.3718000776565,-2.16153189778506));
#6031=CARTESIAN_POINT('Ctrl Pts',(1.98934597530643,36.4968000776565,-1.51515420778634));
#6032=CARTESIAN_POINT('Ctrl Pts',(2.48164942024637,36.6218000776565,-0.868776517787625));
#6033=CARTESIAN_POINT('Ctrl Pts',(2.5,36.7468000776565,-0.0564772772053589));
#6034=CARTESIAN_POINT('Ctrl Pts',(2.51835057975363,36.8718000776565,0.755821963376907));
#6035=CARTESIAN_POINT('Ctrl Pts',(2.05573899656831,36.9968000776565,1.42377205367602));
#6036=CARTESIAN_POINT('Ctrl Pts',(1.593127413383,37.1218000776565,2.09172214397514));
#6037=CARTESIAN_POINT('Ctrl Pts',(0.826255568446133,37.2468000776565,2.3601888522854));
#6038=CARTESIAN_POINT('Ctrl Pts',(0.059383723509268,37.3718000776565,2.62865556059567));
#6039=CARTESIAN_POINT('Ctrl Pts',(-0.718829403428604,37.4968000776565,2.39509372919037));
#6040=CARTESIAN_POINT('Ctrl Pts',(-1.49704253036648,37.6218000776565,2.16153189778506));
#6041=CARTESIAN_POINT('Ctrl Pts',(-1.98934597530643,37.7468000776565,1.51515420778634));
#6042=CARTESIAN_POINT('Ctrl Pts',(-2.48164942024637,37.8718000776565,0.868776517787626));
#6043=CARTESIAN_POINT('Ctrl Pts',(-2.5,37.9968000776565,0.0564772772053586));
#6044=CARTESIAN_POINT('Ctrl Pts',(-2.51835057975363,38.1218000776565,-0.755821963376908));
#6045=CARTESIAN_POINT('Ctrl Pts',(-2.05573899656831,38.2468000776565,-1.42377205367602));
#6046=CARTESIAN_POINT('Ctrl Pts',(-1.593127413383,38.3718000776565,-2.09172214397514));
#6047=CARTESIAN_POINT('Ctrl Pts',(-0.826255568446133,38.4968000776565,-2.3601888522854));
#6048=CARTESIAN_POINT('Ctrl Pts',(-0.0593837235092677,38.6218000776565,
-2.62865556059567));
#6049=CARTESIAN_POINT('Ctrl Pts',(0.718829403428605,38.7468000776565,-2.39509372919037));
#6050=CARTESIAN_POINT('Ctrl Pts',(1.49704253036648,38.8718000776565,-2.16153189778506));
#6051=CARTESIAN_POINT('Ctrl Pts',(1.98934597530643,38.9968000776565,-1.51515420778634));
#6052=CARTESIAN_POINT('Ctrl Pts',(2.48164942024637,39.1218000776565,-0.868776517787625));
#6053=CARTESIAN_POINT('Ctrl Pts',(2.5,39.2468000776565,-0.0564772772053589));
#6054=CARTESIAN_POINT('Ctrl Pts',(2.51835057975363,39.3718000776565,0.755821963376907));
#6055=CARTESIAN_POINT('Ctrl Pts',(2.05573899656831,39.4968000776565,1.42377205367602));
#6056=CARTESIAN_POINT('Ctrl Pts',(1.593127413383,39.6218000776565,2.09172214397514));
#6057=CARTESIAN_POINT('Ctrl Pts',(0.826255568446133,39.7468000776565,2.3601888522854));
#6058=CARTESIAN_POINT('Ctrl Pts',(0.059383723509268,39.8718000776565,2.62865556059567));
#6059=CARTESIAN_POINT('Ctrl Pts',(-0.718829403428604,39.9968000776565,2.39509372919037));
#6060=CARTESIAN_POINT('Ctrl Pts',(-1.49704253036648,40.1218000776565,2.16153189778506));
#6061=CARTESIAN_POINT('Ctrl Pts',(-1.98934597530643,40.2468000776565,1.51515420778634));
#6062=CARTESIAN_POINT('Ctrl Pts',(-2.48164942024637,40.3718000776565,0.868776517787626));
#6063=CARTESIAN_POINT('Ctrl Pts',(-2.5,40.4968000776565,0.0564772772053586));
#6064=CARTESIAN_POINT('Ctrl Pts',(-2.5,14.5031999223435,-0.056477277205306));
#6065=CARTESIAN_POINT('Ctrl Pts',(-2.48164942024639,14.6281999223435,-0.868776517787572));
#6066=CARTESIAN_POINT('Ctrl Pts',(-1.98934597530646,14.7531999223435,-1.5151542077863));
#6067=CARTESIAN_POINT('Ctrl Pts',(-1.49704253036652,14.8781999223435,-2.16153189778503));
#6068=CARTESIAN_POINT('Ctrl Pts',(-0.718829403428655,15.0031999223435,-2.39509372919035));
#6069=CARTESIAN_POINT('Ctrl Pts',(0.0593837235092121,15.1281999223435,-2.62865556059567));
#6070=CARTESIAN_POINT('Ctrl Pts',(0.826255568446083,15.2531999223435,-2.36018885228542));
#6071=CARTESIAN_POINT('Ctrl Pts',(1.59312741338295,15.3781999223435,-2.09172214397517));
#6072=CARTESIAN_POINT('Ctrl Pts',(2.05573899656828,15.5031999223436,-1.42377205367607));
#6073=CARTESIAN_POINT('Ctrl Pts',(2.51835057975361,15.6281999223435,-0.755821963376961));
#6074=CARTESIAN_POINT('Ctrl Pts',(2.5,15.7531999223435,0.0564772772053057));
#6075=CARTESIAN_POINT('Ctrl Pts',(2.48164942024639,15.8781999223435,0.868776517787572));
#6076=CARTESIAN_POINT('Ctrl Pts',(1.98934597530646,16.0031999223435,1.5151542077863));
#6077=CARTESIAN_POINT('Ctrl Pts',(1.49704253036652,16.1281999223435,2.16153189778503));
#6078=CARTESIAN_POINT('Ctrl Pts',(0.718829403428655,16.2531999223435,2.39509372919035));
#6079=CARTESIAN_POINT('Ctrl Pts',(-0.0593837235092117,16.3781999223435,
2.62865556059567));
#6080=CARTESIAN_POINT('Ctrl Pts',(-0.826255568446083,16.5031999223435,2.36018885228542));
#6081=CARTESIAN_POINT('Ctrl Pts',(-1.59312741338295,16.6281999223435,2.09172214397517));
#6082=CARTESIAN_POINT('Ctrl Pts',(-2.05573899656828,16.7531999223435,1.42377205367607));
#6083=CARTESIAN_POINT('Ctrl Pts',(-2.51835057975361,16.8781999223435,0.755821963376961));
#6084=CARTESIAN_POINT('Ctrl Pts',(-2.5,17.0031999223435,-0.056477277205306));
#6085=CARTESIAN_POINT('Ctrl Pts',(-2.48164942024639,17.1281999223435,-0.868776517787572));
#6086=CARTESIAN_POINT('Ctrl Pts',(-1.98934597530646,17.2531999223435,-1.5151542077863));
#6087=CARTESIAN_POINT('Ctrl Pts',(-1.49704253036652,17.3781999223435,-2.16153189778503));
#6088=CARTESIAN_POINT('Ctrl Pts',(-0.718829403428655,17.5031999223435,-2.39509372919035));
#6089=CARTESIAN_POINT('Ctrl Pts',(0.0593837235092121,17.6281999223435,-2.62865556059567));
#6090=CARTESIAN_POINT('Ctrl Pts',(0.826255568446083,17.7531999223435,-2.36018885228542));
#6091=CARTESIAN_POINT('Ctrl Pts',(1.59312741338295,17.8781999223435,-2.09172214397517));
#6092=CARTESIAN_POINT('Ctrl Pts',(2.05573899656828,18.0031999223435,-1.42377205367607));
#6093=CARTESIAN_POINT('Ctrl Pts',(2.51835057975361,18.1281999223435,-0.755821963376961));
#6094=CARTESIAN_POINT('Ctrl Pts',(2.5,18.2531999223435,0.0564772772053057));
#6095=CARTESIAN_POINT('Ctrl Pts',(2.48164942024639,18.3781999223435,0.868776517787572));
#6096=CARTESIAN_POINT('Ctrl Pts',(1.98934597530646,18.5031999223435,1.5151542077863));
#6097=CARTESIAN_POINT('Ctrl Pts',(1.49704253036652,18.6281999223435,2.16153189778503));
#6098=CARTESIAN_POINT('Ctrl Pts',(0.718829403428655,18.7531999223435,2.39509372919035));
#6099=CARTESIAN_POINT('Ctrl Pts',(-0.0593837235092117,18.8781999223435,
2.62865556059567));
#6100=CARTESIAN_POINT('Ctrl Pts',(-0.826255568446083,19.0031999223435,2.36018885228542));
#6101=CARTESIAN_POINT('Ctrl Pts',(-1.59312741338295,19.1281999223435,2.09172214397517));
#6102=CARTESIAN_POINT('Ctrl Pts',(-2.05573899656828,19.2531999223435,1.42377205367607));
#6103=CARTESIAN_POINT('Ctrl Pts',(-2.51835057975361,19.3781999223435,0.755821963376961));
#6104=CARTESIAN_POINT('Ctrl Pts',(-2.5,19.5031999223435,-0.056477277205306));
#6105=CARTESIAN_POINT('Ctrl Pts',(-2.48164942024639,19.6281999223435,-0.868776517787572));
#6106=CARTESIAN_POINT('Ctrl Pts',(-1.98934597530646,19.7531999223435,-1.5151542077863));
#6107=CARTESIAN_POINT('Ctrl Pts',(-1.49704253036652,19.8781999223435,-2.16153189778503));
#6108=CARTESIAN_POINT('Ctrl Pts',(-0.718829403428655,20.0031999223435,-2.39509372919035));
#6109=CARTESIAN_POINT('Ctrl Pts',(0.0593837235092121,20.1281999223436,-2.62865556059567));
#6110=CARTESIAN_POINT('Ctrl Pts',(0.826255568446083,20.2531999223435,-2.36018885228542));
#6111=CARTESIAN_POINT('Ctrl Pts',(1.59312741338295,20.3781999223435,-2.09172214397517));
#6112=CARTESIAN_POINT('Ctrl Pts',(2.05573899656828,20.5031999223436,-1.42377205367607));
#6113=CARTESIAN_POINT('Ctrl Pts',(2.51835057975361,20.6281999223435,-0.755821963376961));
#6114=CARTESIAN_POINT('Ctrl Pts',(2.5,20.7531999223436,0.0564772772053057));
#6115=CARTESIAN_POINT('Ctrl Pts',(2.48164942024639,20.8781999223436,0.868776517787572));
#6116=CARTESIAN_POINT('Ctrl Pts',(1.98934597530646,21.0031999223435,1.5151542077863));
#6117=CARTESIAN_POINT('Ctrl Pts',(1.49704253036652,21.1281999223435,2.16153189778503));
#6118=CARTESIAN_POINT('Ctrl Pts',(0.718829403428655,21.2531999223435,2.39509372919035));
#6119=CARTESIAN_POINT('Ctrl Pts',(-0.0593837235092117,21.3781999223435,
2.62865556059567));
#6120=CARTESIAN_POINT('Ctrl Pts',(-0.826255568446083,21.5031999223435,2.36018885228542));
#6121=CARTESIAN_POINT('Ctrl Pts',(-1.59312741338295,21.6281999223435,2.09172214397517));
#6122=CARTESIAN_POINT('Ctrl Pts',(-2.05573899656828,21.7531999223435,1.42377205367607));
#6123=CARTESIAN_POINT('Ctrl Pts',(-2.51835057975361,21.8781999223435,0.755821963376961));
#6124=CARTESIAN_POINT('Ctrl Pts',(-2.5,22.0031999223436,-0.056477277205306));
#6125=CARTESIAN_POINT('Ctrl Pts',(-2.48164942024639,22.1281999223435,-0.868776517787572));
#6126=CARTESIAN_POINT('Ctrl Pts',(-1.98934597530646,22.2531999223435,-1.5151542077863));
#6127=CARTESIAN_POINT('Ctrl Pts',(-1.49704253036652,22.3781999223435,-2.16153189778503));
#6128=CARTESIAN_POINT('Ctrl Pts',(-0.718829403428655,22.5031999223435,-2.39509372919035));
#6129=CARTESIAN_POINT('Ctrl Pts',(0.0593837235092121,22.6281999223436,-2.62865556059567));
#6130=CARTESIAN_POINT('Ctrl Pts',(0.826255568446083,22.7531999223435,-2.36018885228542));
#6131=CARTESIAN_POINT('Ctrl Pts',(1.59312741338295,22.8781999223435,-2.09172214397517));
#6132=CARTESIAN_POINT('Ctrl Pts',(2.05573899656828,23.0031999223435,-1.42377205367607));
#6133=CARTESIAN_POINT('Ctrl Pts',(2.51835057975361,23.1281999223435,-0.755821963376961));
#6134=CARTESIAN_POINT('Ctrl Pts',(2.5,23.2531999223436,0.0564772772053057));
#6135=CARTESIAN_POINT('Ctrl Pts',(2.48164942024639,23.3781999223435,0.868776517787572));
#6136=CARTESIAN_POINT('Ctrl Pts',(1.98934597530646,23.5031999223436,1.5151542077863));
#6137=CARTESIAN_POINT('Ctrl Pts',(1.49704253036652,23.6281999223435,2.16153189778503));
#6138=CARTESIAN_POINT('Ctrl Pts',(0.718829403428655,23.7531999223435,2.39509372919035));
#6139=CARTESIAN_POINT('Ctrl Pts',(-0.0593837235092117,23.8781999223435,
2.62865556059567));
#6140=CARTESIAN_POINT('Ctrl Pts',(-0.826255568446083,24.0031999223435,2.36018885228542));
#6141=CARTESIAN_POINT('Ctrl Pts',(-1.59312741338295,24.1281999223435,2.09172214397517));
#6142=CARTESIAN_POINT('Ctrl Pts',(-2.05573899656828,24.2531999223435,1.42377205367607));
#6143=CARTESIAN_POINT('Ctrl Pts',(-2.51835057975361,24.3781999223435,0.755821963376961));
#6144=CARTESIAN_POINT('Ctrl Pts',(-2.5,24.5031999223436,-0.056477277205306));
#6145=CARTESIAN_POINT('Ctrl Pts',(-2.48164942024639,24.6281999223435,-0.868776517787572));
#6146=CARTESIAN_POINT('Ctrl Pts',(-1.98934597530646,24.7531999223435,-1.5151542077863));
#6147=CARTESIAN_POINT('Ctrl Pts',(-1.49704253036652,24.8781999223436,-2.16153189778503));
#6148=CARTESIAN_POINT('Ctrl Pts',(-0.718829403428655,25.0031999223435,-2.39509372919035));
#6149=CARTESIAN_POINT('Ctrl Pts',(0.0593837235092121,25.1281999223435,-2.62865556059567));
#6150=CARTESIAN_POINT('Ctrl Pts',(0.826255568446083,25.2531999223435,-2.36018885228542));
#6151=CARTESIAN_POINT('Ctrl Pts',(1.59312741338295,25.3781999223435,-2.09172214397517));
#6152=CARTESIAN_POINT('Ctrl Pts',(2.05573899656828,25.5031999223435,-1.42377205367607));
#6153=CARTESIAN_POINT('Ctrl Pts',(2.51835057975361,25.6281999223435,-0.755821963376961));
#6154=CARTESIAN_POINT('Ctrl Pts',(2.5,25.7531999223436,0.0564772772053057));
#6155=CARTESIAN_POINT('Ctrl Pts',(2.48164942024639,25.8781999223436,0.868776517787572));
#6156=CARTESIAN_POINT('Ctrl Pts',(1.98934597530646,26.0031999223435,1.5151542077863));
#6157=CARTESIAN_POINT('Ctrl Pts',(1.49704253036652,26.1281999223435,2.16153189778503));
#6158=CARTESIAN_POINT('Ctrl Pts',(0.718829403428655,26.2531999223435,2.39509372919035));
#6159=CARTESIAN_POINT('Ctrl Pts',(-0.0593837235092117,26.3781999223436,
2.62865556059567));
#6160=CARTESIAN_POINT('Ctrl Pts',(-0.826255568446083,26.5031999223435,2.36018885228542));
#6161=CARTESIAN_POINT('Ctrl Pts',(-1.59312741338295,26.6281999223435,2.09172214397517));
#6162=CARTESIAN_POINT('Ctrl Pts',(-2.05573899656828,26.7531999223436,1.42377205367607));
#6163=CARTESIAN_POINT('Ctrl Pts',(-2.51835057975361,26.8781999223435,0.755821963376961));
#6164=CARTESIAN_POINT('Ctrl Pts',(-2.5,27.0031999223436,-0.056477277205306));
#6165=CARTESIAN_POINT('Ctrl Pts',(-2.48164942024639,27.1281999223436,-0.868776517787572));
#6166=CARTESIAN_POINT('Ctrl Pts',(-1.98934597530646,27.2531999223435,-1.5151542077863));
#6167=CARTESIAN_POINT('Ctrl Pts',(-1.49704253036652,27.3781999223436,-2.16153189778503));
#6168=CARTESIAN_POINT('Ctrl Pts',(-0.718829403428655,27.5031999223435,-2.39509372919035));
#6169=CARTESIAN_POINT('Ctrl Pts',(0.0593837235092121,27.6281999223435,-2.62865556059567));
#6170=CARTESIAN_POINT('Ctrl Pts',(0.826255568446083,27.7531999223436,-2.36018885228542));
#6171=CARTESIAN_POINT('Ctrl Pts',(1.59312741338295,27.8781999223436,-2.09172214397517));
#6172=CARTESIAN_POINT('Ctrl Pts',(2.05573899656828,28.0031999223436,-1.42377205367607));
#6173=CARTESIAN_POINT('Ctrl Pts',(2.51835057975361,28.1281999223436,-0.755821963376961));
#6174=CARTESIAN_POINT('Ctrl Pts',(2.5,28.2531999223436,0.0564772772053057));
#6175=CARTESIAN_POINT('Ctrl Pts',(2.48164942024639,28.3781999223436,0.868776517787572));
#6176=CARTESIAN_POINT('Ctrl Pts',(1.98934597530646,28.5031999223436,1.5151542077863));
#6177=CARTESIAN_POINT('Ctrl Pts',(1.49704253036652,28.6281999223436,2.16153189778503));
#6178=CARTESIAN_POINT('Ctrl Pts',(0.718829403428655,28.7531999223435,2.39509372919035));
#6179=CARTESIAN_POINT('Ctrl Pts',(-0.0593837235092117,28.8781999223435,
2.62865556059567));
#6180=CARTESIAN_POINT('Ctrl Pts',(-0.826255568446083,29.0031999223436,2.36018885228542));
#6181=CARTESIAN_POINT('Ctrl Pts',(-1.59312741338295,29.1281999223435,2.09172214397517));
#6182=CARTESIAN_POINT('Ctrl Pts',(-2.05573899656828,29.2531999223436,1.42377205367607));
#6183=CARTESIAN_POINT('Ctrl Pts',(-2.51835057975361,29.3781999223436,0.755821963376961));
#6184=CARTESIAN_POINT('Ctrl Pts',(-2.5,29.5031999223436,-0.056477277205306));
#6185=CARTESIAN_POINT('Ctrl Pts',(-2.48164942024639,29.6281999223435,-0.868776517787572));
#6186=CARTESIAN_POINT('Ctrl Pts',(-1.98934597530646,29.7531999223435,-1.5151542077863));
#6187=CARTESIAN_POINT('Ctrl Pts',(-1.49704253036652,29.8781999223435,-2.16153189778503));
#6188=CARTESIAN_POINT('Ctrl Pts',(-0.718829403428655,30.0031999223435,-2.39509372919035));
#6189=CARTESIAN_POINT('Ctrl Pts',(0.0593837235092121,30.1281999223435,-2.62865556059567));
#6190=CARTESIAN_POINT('Ctrl Pts',(0.826255568446083,30.2531999223435,-2.36018885228542));
#6191=CARTESIAN_POINT('Ctrl Pts',(1.59312741338295,30.3781999223435,-2.09172214397517));
#6192=CARTESIAN_POINT('Ctrl Pts',(2.05573899656828,30.5031999223436,-1.42377205367607));
#6193=CARTESIAN_POINT('Ctrl Pts',(2.51835057975361,30.6281999223436,-0.755821963376961));
#6194=CARTESIAN_POINT('Ctrl Pts',(2.5,30.7531999223435,0.0564772772053057));
#6195=CARTESIAN_POINT('Ctrl Pts',(2.48164942024639,30.8781999223435,0.868776517787572));
#6196=CARTESIAN_POINT('Ctrl Pts',(1.98934597530646,31.0031999223436,1.5151542077863));
#6197=CARTESIAN_POINT('Ctrl Pts',(1.49704253036652,31.1281999223435,2.16153189778503));
#6198=CARTESIAN_POINT('Ctrl Pts',(0.718829403428655,31.2531999223435,2.39509372919035));
#6199=CARTESIAN_POINT('Ctrl Pts',(-0.0593837235092117,31.3781999223435,
2.62865556059567));
#6200=CARTESIAN_POINT('Ctrl Pts',(-0.826255568446083,31.5031999223435,2.36018885228542));
#6201=CARTESIAN_POINT('Ctrl Pts',(-1.59312741338295,31.6281999223435,2.09172214397517));
#6202=CARTESIAN_POINT('Ctrl Pts',(-2.05573899656828,31.7531999223436,1.42377205367607));
#6203=CARTESIAN_POINT('Ctrl Pts',(-2.51835057975361,31.8781999223435,0.755821963376961));
#6204=CARTESIAN_POINT('Ctrl Pts',(-2.5,32.0031999223435,-0.056477277205306));
#6205=CARTESIAN_POINT('Ctrl Pts',(-2.48164942024639,32.1281999223435,-0.868776517787572));
#6206=CARTESIAN_POINT('Ctrl Pts',(-1.98934597530646,32.2531999223435,-1.5151542077863));
#6207=CARTESIAN_POINT('Ctrl Pts',(-1.49704253036652,32.3781999223435,-2.16153189778503));
#6208=CARTESIAN_POINT('Ctrl Pts',(-0.718829403428655,32.5031999223435,-2.39509372919035));
#6209=CARTESIAN_POINT('Ctrl Pts',(0.0593837235092121,32.6281999223435,-2.62865556059567));
#6210=CARTESIAN_POINT('Ctrl Pts',(0.826255568446083,32.7531999223435,-2.36018885228542));
#6211=CARTESIAN_POINT('Ctrl Pts',(1.59312741338295,32.8781999223435,-2.09172214397517));
#6212=CARTESIAN_POINT('Ctrl Pts',(2.05573899656828,33.0031999223436,-1.42377205367607));
#6213=CARTESIAN_POINT('Ctrl Pts',(2.51835057975361,33.1281999223435,-0.755821963376961));
#6214=CARTESIAN_POINT('Ctrl Pts',(2.5,33.2531999223435,0.0564772772053057));
#6215=CARTESIAN_POINT('Ctrl Pts',(2.48164942024639,33.3781999223435,0.868776517787572));
#6216=CARTESIAN_POINT('Ctrl Pts',(1.98934597530646,33.5031999223435,1.5151542077863));
#6217=CARTESIAN_POINT('Ctrl Pts',(1.49704253036652,33.6281999223436,2.16153189778503));
#6218=CARTESIAN_POINT('Ctrl Pts',(0.718829403428655,33.7531999223435,2.39509372919035));
#6219=CARTESIAN_POINT('Ctrl Pts',(-0.0593837235092117,33.8781999223435,
2.62865556059567));
#6220=CARTESIAN_POINT('Ctrl Pts',(-0.826255568446083,34.0031999223435,2.36018885228542));
#6221=CARTESIAN_POINT('Ctrl Pts',(-1.59312741338295,34.1281999223435,2.09172214397517));
#6222=CARTESIAN_POINT('Ctrl Pts',(-2.05573899656828,34.2531999223435,1.42377205367607));
#6223=CARTESIAN_POINT('Ctrl Pts',(-2.51835057975361,34.3781999223435,0.755821963376961));
#6224=CARTESIAN_POINT('Ctrl Pts',(-2.5,34.5031999223435,-0.056477277205306));
#6225=CARTESIAN_POINT('Ctrl Pts',(-2.48164942024639,34.6281999223435,-0.868776517787572));
#6226=CARTESIAN_POINT('Ctrl Pts',(-1.98934597530646,34.7531999223435,-1.5151542077863));
#6227=CARTESIAN_POINT('Ctrl Pts',(-1.49704253036652,34.8781999223436,-2.16153189778503));
#6228=CARTESIAN_POINT('Ctrl Pts',(-0.718829403428655,35.0031999223435,-2.39509372919035));
#6229=CARTESIAN_POINT('Ctrl Pts',(0.0593837235092121,35.1281999223435,-2.62865556059567));
#6230=CARTESIAN_POINT('Ctrl Pts',(0.826255568446083,35.2531999223435,-2.36018885228542));
#6231=CARTESIAN_POINT('Ctrl Pts',(1.59312741338295,35.3781999223435,-2.09172214397517));
#6232=CARTESIAN_POINT('Ctrl Pts',(2.05573899656828,35.5031999223436,-1.42377205367607));
#6233=CARTESIAN_POINT('Ctrl Pts',(2.51835057975361,35.6281999223435,-0.755821963376961));
#6234=CARTESIAN_POINT('Ctrl Pts',(2.5,35.7531999223435,0.0564772772053057));
#6235=CARTESIAN_POINT('Ctrl Pts',(2.48164942024639,35.8781999223435,0.868776517787572));
#6236=CARTESIAN_POINT('Ctrl Pts',(1.98934597530646,36.0031999223435,1.5151542077863));
#6237=CARTESIAN_POINT('Ctrl Pts',(1.49704253036652,36.1281999223436,2.16153189778503));
#6238=CARTESIAN_POINT('Ctrl Pts',(0.718829403428655,36.2531999223435,2.39509372919035));
#6239=CARTESIAN_POINT('Ctrl Pts',(-0.0593837235092117,36.3781999223435,
2.62865556059567));
#6240=CARTESIAN_POINT('Ctrl Pts',(-0.826255568446083,36.5031999223435,2.36018885228542));
#6241=CARTESIAN_POINT('Ctrl Pts',(-1.59312741338295,36.6281999223435,2.09172214397517));
#6242=CARTESIAN_POINT('Ctrl Pts',(-2.05573899656828,36.7531999223436,1.42377205367607));
#6243=CARTESIAN_POINT('Ctrl Pts',(-2.51835057975361,36.8781999223435,0.755821963376961));
#6244=CARTESIAN_POINT('Ctrl Pts',(-2.5,37.0031999223435,-0.056477277205306));
#6245=CARTESIAN_POINT('Ctrl Pts',(-2.48164942024639,37.1281999223435,-0.868776517787572));
#6246=CARTESIAN_POINT('Ctrl Pts',(-1.98934597530646,37.2531999223435,-1.5151542077863));
#6247=CARTESIAN_POINT('Ctrl Pts',(-1.49704253036652,37.3781999223436,-2.16153189778503));
#6248=CARTESIAN_POINT('Ctrl Pts',(-0.718829403428655,37.5031999223435,-2.39509372919035));
#6249=CARTESIAN_POINT('Ctrl Pts',(0.0593837235092121,37.6281999223435,-2.62865556059567));
#6250=CARTESIAN_POINT('Ctrl Pts',(0.826255568446083,37.7531999223435,-2.36018885228542));
#6251=CARTESIAN_POINT('Ctrl Pts',(1.59312741338295,37.8781999223435,-2.09172214397517));
#6252=CARTESIAN_POINT('Ctrl Pts',(2.05573899656828,38.0031999223435,-1.42377205367607));
#6253=CARTESIAN_POINT('Ctrl Pts',(2.51835057975361,38.1281999223435,-0.755821963376961));
#6254=CARTESIAN_POINT('Ctrl Pts',(2.5,38.2531999223435,0.0564772772053057));
#6255=CARTESIAN_POINT('Ctrl Pts',(2.48164942024639,38.3781999223435,0.868776517787572));
#6256=CARTESIAN_POINT('Ctrl Pts',(1.98934597530646,38.5031999223435,1.5151542077863));
#6257=CARTESIAN_POINT('Ctrl Pts',(1.49704253036652,38.6281999223436,2.16153189778503));
#6258=CARTESIAN_POINT('Ctrl Pts',(0.718829403428655,38.7531999223435,2.39509372919035));
#6259=CARTESIAN_POINT('Ctrl Pts',(-0.0593837235092117,38.8781999223435,
2.62865556059567));
#6260=CARTESIAN_POINT('Ctrl Pts',(-0.826255568446083,39.0031999223436,2.36018885228542));
#6261=CARTESIAN_POINT('Ctrl Pts',(-1.59312741338295,39.1281999223435,2.09172214397517));
#6262=CARTESIAN_POINT('Ctrl Pts',(-2.05573899656828,39.2531999223436,1.42377205367607));
#6263=CARTESIAN_POINT('Ctrl Pts',(-2.51835057975361,39.3781999223435,0.755821963376961));
#6264=CARTESIAN_POINT('Ctrl Pts',(-2.5,39.5031999223436,-0.056477277205306));
#6265=CARTESIAN_POINT('Ctrl Pts',(-3.5,14.5031999223435,-0.0564772772052956));
#6266=CARTESIAN_POINT('Ctrl Pts',(-3.48164942024639,14.6281999223435,-1.19369621402047));
#6267=CARTESIAN_POINT('Ctrl Pts',(-2.79836296968141,14.7531999223435,-2.10293946007877));
#6268=CARTESIAN_POINT('Ctrl Pts',(-2.11507651911643,14.8781999223435,-3.01218270613706));
#6269=CARTESIAN_POINT('Ctrl Pts',(-1.02784639780361,15.0031999223435,-3.3461502454855));
#6270=CARTESIAN_POINT('Ctrl Pts',(0.0593837235092011,15.1281999223435,-3.68011778483394));
#6271=CARTESIAN_POINT('Ctrl Pts',(1.13527256282102,15.2531999223435,-3.31124536858058));
#6272=CARTESIAN_POINT('Ctrl Pts',(2.21116140213284,15.3781999223435,-2.94237295232722));
#6273=CARTESIAN_POINT('Ctrl Pts',(2.86475599094322,15.5031999223435,-2.01155730596855));
#6274=CARTESIAN_POINT('Ctrl Pts',(3.51835057975361,15.6281999223435,-1.08074165960988));
#6275=CARTESIAN_POINT('Ctrl Pts',(3.5,15.7531999223435,0.0564772772052952));
#6276=CARTESIAN_POINT('Ctrl Pts',(3.48164942024639,15.8781999223435,1.19369621402047));
#6277=CARTESIAN_POINT('Ctrl Pts',(2.79836296968141,16.0031999223435,2.10293946007876));
#6278=CARTESIAN_POINT('Ctrl Pts',(2.11507651911643,16.1281999223435,3.01218270613706));
#6279=CARTESIAN_POINT('Ctrl Pts',(1.02784639780361,16.2531999223435,3.3461502454855));
#6280=CARTESIAN_POINT('Ctrl Pts',(-0.0593837235092006,16.3781999223435,
3.68011778483394));
#6281=CARTESIAN_POINT('Ctrl Pts',(-1.13527256282102,16.5031999223435,3.31124536858058));
#6282=CARTESIAN_POINT('Ctrl Pts',(-2.21116140213284,16.6281999223435,2.94237295232722));
#6283=CARTESIAN_POINT('Ctrl Pts',(-2.86475599094322,16.7531999223435,2.01155730596855));
#6284=CARTESIAN_POINT('Ctrl Pts',(-3.51835057975361,16.8781999223435,1.08074165960988));
#6285=CARTESIAN_POINT('Ctrl Pts',(-3.5,17.0031999223435,-0.0564772772052956));
#6286=CARTESIAN_POINT('Ctrl Pts',(-3.48164942024639,17.1281999223435,-1.19369621402047));
#6287=CARTESIAN_POINT('Ctrl Pts',(-2.79836296968141,17.2531999223435,-2.10293946007877));
#6288=CARTESIAN_POINT('Ctrl Pts',(-2.11507651911643,17.3781999223435,-3.01218270613706));
#6289=CARTESIAN_POINT('Ctrl Pts',(-1.02784639780361,17.5031999223435,-3.3461502454855));
#6290=CARTESIAN_POINT('Ctrl Pts',(0.0593837235092011,17.6281999223435,-3.68011778483394));
#6291=CARTESIAN_POINT('Ctrl Pts',(1.13527256282102,17.7531999223435,-3.31124536858058));
#6292=CARTESIAN_POINT('Ctrl Pts',(2.21116140213284,17.8781999223435,-2.94237295232722));
#6293=CARTESIAN_POINT('Ctrl Pts',(2.86475599094322,18.0031999223435,-2.01155730596855));
#6294=CARTESIAN_POINT('Ctrl Pts',(3.51835057975361,18.1281999223435,-1.08074165960988));
#6295=CARTESIAN_POINT('Ctrl Pts',(3.5,18.2531999223435,0.0564772772052952));
#6296=CARTESIAN_POINT('Ctrl Pts',(3.48164942024639,18.3781999223435,1.19369621402047));
#6297=CARTESIAN_POINT('Ctrl Pts',(2.79836296968141,18.5031999223435,2.10293946007876));
#6298=CARTESIAN_POINT('Ctrl Pts',(2.11507651911643,18.6281999223435,3.01218270613706));
#6299=CARTESIAN_POINT('Ctrl Pts',(1.02784639780361,18.7531999223435,3.3461502454855));
#6300=CARTESIAN_POINT('Ctrl Pts',(-0.0593837235092006,18.8781999223435,
3.68011778483394));
#6301=CARTESIAN_POINT('Ctrl Pts',(-1.13527256282102,19.0031999223435,3.31124536858058));
#6302=CARTESIAN_POINT('Ctrl Pts',(-2.21116140213284,19.1281999223435,2.94237295232722));
#6303=CARTESIAN_POINT('Ctrl Pts',(-2.86475599094322,19.2531999223435,2.01155730596855));
#6304=CARTESIAN_POINT('Ctrl Pts',(-3.51835057975361,19.3781999223435,1.08074165960988));
#6305=CARTESIAN_POINT('Ctrl Pts',(-3.5,19.5031999223435,-0.0564772772052956));
#6306=CARTESIAN_POINT('Ctrl Pts',(-3.48164942024639,19.6281999223435,-1.19369621402047));
#6307=CARTESIAN_POINT('Ctrl Pts',(-2.79836296968141,19.7531999223435,-2.10293946007877));
#6308=CARTESIAN_POINT('Ctrl Pts',(-2.11507651911643,19.8781999223435,-3.01218270613706));
#6309=CARTESIAN_POINT('Ctrl Pts',(-1.02784639780361,20.0031999223435,-3.3461502454855));
#6310=CARTESIAN_POINT('Ctrl Pts',(0.0593837235092011,20.1281999223435,-3.68011778483394));
#6311=CARTESIAN_POINT('Ctrl Pts',(1.13527256282102,20.2531999223435,-3.31124536858058));
#6312=CARTESIAN_POINT('Ctrl Pts',(2.21116140213284,20.3781999223435,-2.94237295232722));
#6313=CARTESIAN_POINT('Ctrl Pts',(2.86475599094322,20.5031999223435,-2.01155730596855));
#6314=CARTESIAN_POINT('Ctrl Pts',(3.51835057975361,20.6281999223435,-1.08074165960988));
#6315=CARTESIAN_POINT('Ctrl Pts',(3.5,20.7531999223435,0.0564772772052952));
#6316=CARTESIAN_POINT('Ctrl Pts',(3.48164942024639,20.8781999223435,1.19369621402047));
#6317=CARTESIAN_POINT('Ctrl Pts',(2.79836296968141,21.0031999223435,2.10293946007876));
#6318=CARTESIAN_POINT('Ctrl Pts',(2.11507651911643,21.1281999223435,3.01218270613706));
#6319=CARTESIAN_POINT('Ctrl Pts',(1.02784639780361,21.2531999223435,3.3461502454855));
#6320=CARTESIAN_POINT('Ctrl Pts',(-0.0593837235092006,21.3781999223435,
3.68011778483394));
#6321=CARTESIAN_POINT('Ctrl Pts',(-1.13527256282102,21.5031999223435,3.31124536858058));
#6322=CARTESIAN_POINT('Ctrl Pts',(-2.21116140213284,21.6281999223435,2.94237295232722));
#6323=CARTESIAN_POINT('Ctrl Pts',(-2.86475599094322,21.7531999223435,2.01155730596855));
#6324=CARTESIAN_POINT('Ctrl Pts',(-3.51835057975361,21.8781999223435,1.08074165960988));
#6325=CARTESIAN_POINT('Ctrl Pts',(-3.5,22.0031999223435,-0.0564772772052956));
#6326=CARTESIAN_POINT('Ctrl Pts',(-3.48164942024639,22.1281999223435,-1.19369621402047));
#6327=CARTESIAN_POINT('Ctrl Pts',(-2.79836296968141,22.2531999223435,-2.10293946007877));
#6328=CARTESIAN_POINT('Ctrl Pts',(-2.11507651911643,22.3781999223435,-3.01218270613706));
#6329=CARTESIAN_POINT('Ctrl Pts',(-1.02784639780361,22.5031999223435,-3.3461502454855));
#6330=CARTESIAN_POINT('Ctrl Pts',(0.0593837235092011,22.6281999223435,-3.68011778483394));
#6331=CARTESIAN_POINT('Ctrl Pts',(1.13527256282102,22.7531999223435,-3.31124536858058));
#6332=CARTESIAN_POINT('Ctrl Pts',(2.21116140213284,22.8781999223435,-2.94237295232722));
#6333=CARTESIAN_POINT('Ctrl Pts',(2.86475599094322,23.0031999223435,-2.01155730596855));
#6334=CARTESIAN_POINT('Ctrl Pts',(3.51835057975361,23.1281999223435,-1.08074165960988));
#6335=CARTESIAN_POINT('Ctrl Pts',(3.5,23.2531999223435,0.0564772772052952));
#6336=CARTESIAN_POINT('Ctrl Pts',(3.48164942024639,23.3781999223435,1.19369621402047));
#6337=CARTESIAN_POINT('Ctrl Pts',(2.79836296968141,23.5031999223435,2.10293946007876));
#6338=CARTESIAN_POINT('Ctrl Pts',(2.11507651911643,23.6281999223435,3.01218270613706));
#6339=CARTESIAN_POINT('Ctrl Pts',(1.02784639780361,23.7531999223435,3.3461502454855));
#6340=CARTESIAN_POINT('Ctrl Pts',(-0.0593837235092006,23.8781999223435,
3.68011778483394));
#6341=CARTESIAN_POINT('Ctrl Pts',(-1.13527256282102,24.0031999223435,3.31124536858058));
#6342=CARTESIAN_POINT('Ctrl Pts',(-2.21116140213284,24.1281999223435,2.94237295232722));
#6343=CARTESIAN_POINT('Ctrl Pts',(-2.86475599094322,24.2531999223435,2.01155730596855));
#6344=CARTESIAN_POINT('Ctrl Pts',(-3.51835057975361,24.3781999223435,1.08074165960988));
#6345=CARTESIAN_POINT('Ctrl Pts',(-3.5,24.5031999223435,-0.0564772772052956));
#6346=CARTESIAN_POINT('Ctrl Pts',(-3.48164942024639,24.6281999223435,-1.19369621402047));
#6347=CARTESIAN_POINT('Ctrl Pts',(-2.79836296968141,24.7531999223435,-2.10293946007877));
#6348=CARTESIAN_POINT('Ctrl Pts',(-2.11507651911643,24.8781999223436,-3.01218270613706));
#6349=CARTESIAN_POINT('Ctrl Pts',(-1.02784639780361,25.0031999223435,-3.3461502454855));
#6350=CARTESIAN_POINT('Ctrl Pts',(0.0593837235092011,25.1281999223435,-3.68011778483394));
#6351=CARTESIAN_POINT('Ctrl Pts',(1.13527256282102,25.2531999223435,-3.31124536858058));
#6352=CARTESIAN_POINT('Ctrl Pts',(2.21116140213284,25.3781999223435,-2.94237295232722));
#6353=CARTESIAN_POINT('Ctrl Pts',(2.86475599094322,25.5031999223436,-2.01155730596855));
#6354=CARTESIAN_POINT('Ctrl Pts',(3.51835057975361,25.6281999223435,-1.08074165960988));
#6355=CARTESIAN_POINT('Ctrl Pts',(3.5,25.7531999223436,0.0564772772052952));
#6356=CARTESIAN_POINT('Ctrl Pts',(3.48164942024639,25.8781999223435,1.19369621402047));
#6357=CARTESIAN_POINT('Ctrl Pts',(2.79836296968141,26.0031999223435,2.10293946007876));
#6358=CARTESIAN_POINT('Ctrl Pts',(2.11507651911643,26.1281999223436,3.01218270613706));
#6359=CARTESIAN_POINT('Ctrl Pts',(1.02784639780361,26.2531999223435,3.3461502454855));
#6360=CARTESIAN_POINT('Ctrl Pts',(-0.0593837235092006,26.3781999223435,
3.68011778483394));
#6361=CARTESIAN_POINT('Ctrl Pts',(-1.13527256282102,26.5031999223435,3.31124536858058));
#6362=CARTESIAN_POINT('Ctrl Pts',(-2.21116140213284,26.6281999223435,2.94237295232722));
#6363=CARTESIAN_POINT('Ctrl Pts',(-2.86475599094322,26.7531999223436,2.01155730596855));
#6364=CARTESIAN_POINT('Ctrl Pts',(-3.51835057975361,26.8781999223435,1.08074165960988));
#6365=CARTESIAN_POINT('Ctrl Pts',(-3.5,27.0031999223436,-0.0564772772052956));
#6366=CARTESIAN_POINT('Ctrl Pts',(-3.48164942024639,27.1281999223435,-1.19369621402047));
#6367=CARTESIAN_POINT('Ctrl Pts',(-2.79836296968141,27.2531999223435,-2.10293946007877));
#6368=CARTESIAN_POINT('Ctrl Pts',(-2.11507651911643,27.3781999223436,-3.01218270613706));
#6369=CARTESIAN_POINT('Ctrl Pts',(-1.02784639780361,27.5031999223435,-3.3461502454855));
#6370=CARTESIAN_POINT('Ctrl Pts',(0.0593837235092011,27.6281999223435,-3.68011778483394));
#6371=CARTESIAN_POINT('Ctrl Pts',(1.13527256282102,27.7531999223435,-3.31124536858058));
#6372=CARTESIAN_POINT('Ctrl Pts',(2.21116140213284,27.8781999223435,-2.94237295232722));
#6373=CARTESIAN_POINT('Ctrl Pts',(2.86475599094322,28.0031999223435,-2.01155730596855));
#6374=CARTESIAN_POINT('Ctrl Pts',(3.51835057975361,28.1281999223435,-1.08074165960988));
#6375=CARTESIAN_POINT('Ctrl Pts',(3.5,28.2531999223435,0.0564772772052952));
#6376=CARTESIAN_POINT('Ctrl Pts',(3.48164942024639,28.3781999223435,1.19369621402047));
#6377=CARTESIAN_POINT('Ctrl Pts',(2.79836296968141,28.5031999223435,2.10293946007876));
#6378=CARTESIAN_POINT('Ctrl Pts',(2.11507651911643,28.6281999223435,3.01218270613706));
#6379=CARTESIAN_POINT('Ctrl Pts',(1.02784639780361,28.7531999223435,3.3461502454855));
#6380=CARTESIAN_POINT('Ctrl Pts',(-0.0593837235092006,28.8781999223435,
3.68011778483394));
#6381=CARTESIAN_POINT('Ctrl Pts',(-1.13527256282102,29.0031999223435,3.31124536858058));
#6382=CARTESIAN_POINT('Ctrl Pts',(-2.21116140213284,29.1281999223435,2.94237295232722));
#6383=CARTESIAN_POINT('Ctrl Pts',(-2.86475599094322,29.2531999223435,2.01155730596855));
#6384=CARTESIAN_POINT('Ctrl Pts',(-3.51835057975361,29.3781999223435,1.08074165960988));
#6385=CARTESIAN_POINT('Ctrl Pts',(-3.5,29.5031999223435,-0.0564772772052956));
#6386=CARTESIAN_POINT('Ctrl Pts',(-3.48164942024639,29.6281999223435,-1.19369621402047));
#6387=CARTESIAN_POINT('Ctrl Pts',(-2.79836296968141,29.7531999223435,-2.10293946007877));
#6388=CARTESIAN_POINT('Ctrl Pts',(-2.11507651911643,29.8781999223435,-3.01218270613706));
#6389=CARTESIAN_POINT('Ctrl Pts',(-1.02784639780361,30.0031999223435,-3.3461502454855));
#6390=CARTESIAN_POINT('Ctrl Pts',(0.0593837235092011,30.1281999223435,-3.68011778483394));
#6391=CARTESIAN_POINT('Ctrl Pts',(1.13527256282102,30.2531999223435,-3.31124536858058));
#6392=CARTESIAN_POINT('Ctrl Pts',(2.21116140213284,30.3781999223435,-2.94237295232722));
#6393=CARTESIAN_POINT('Ctrl Pts',(2.86475599094322,30.5031999223435,-2.01155730596855));
#6394=CARTESIAN_POINT('Ctrl Pts',(3.51835057975361,30.6281999223435,-1.08074165960988));
#6395=CARTESIAN_POINT('Ctrl Pts',(3.5,30.7531999223435,0.0564772772052952));
#6396=CARTESIAN_POINT('Ctrl Pts',(3.48164942024639,30.8781999223435,1.19369621402047));
#6397=CARTESIAN_POINT('Ctrl Pts',(2.79836296968141,31.0031999223435,2.10293946007876));
#6398=CARTESIAN_POINT('Ctrl Pts',(2.11507651911643,31.1281999223435,3.01218270613706));
#6399=CARTESIAN_POINT('Ctrl Pts',(1.02784639780361,31.2531999223435,3.3461502454855));
#6400=CARTESIAN_POINT('Ctrl Pts',(-0.0593837235092006,31.3781999223435,
3.68011778483394));
#6401=CARTESIAN_POINT('Ctrl Pts',(-1.13527256282102,31.5031999223435,3.31124536858058));
#6402=CARTESIAN_POINT('Ctrl Pts',(-2.21116140213284,31.6281999223435,2.94237295232722));
#6403=CARTESIAN_POINT('Ctrl Pts',(-2.86475599094322,31.7531999223435,2.01155730596855));
#6404=CARTESIAN_POINT('Ctrl Pts',(-3.51835057975361,31.8781999223435,1.08074165960988));
#6405=CARTESIAN_POINT('Ctrl Pts',(-3.5,32.0031999223435,-0.0564772772052956));
#6406=CARTESIAN_POINT('Ctrl Pts',(-3.48164942024639,32.1281999223435,-1.19369621402047));
#6407=CARTESIAN_POINT('Ctrl Pts',(-2.79836296968141,32.2531999223435,-2.10293946007877));
#6408=CARTESIAN_POINT('Ctrl Pts',(-2.11507651911643,32.3781999223436,-3.01218270613706));
#6409=CARTESIAN_POINT('Ctrl Pts',(-1.02784639780361,32.5031999223435,-3.3461502454855));
#6410=CARTESIAN_POINT('Ctrl Pts',(0.0593837235092011,32.6281999223435,-3.68011778483394));
#6411=CARTESIAN_POINT('Ctrl Pts',(1.13527256282102,32.7531999223435,-3.31124536858058));
#6412=CARTESIAN_POINT('Ctrl Pts',(2.21116140213284,32.8781999223435,-2.94237295232722));
#6413=CARTESIAN_POINT('Ctrl Pts',(2.86475599094322,33.0031999223436,-2.01155730596855));
#6414=CARTESIAN_POINT('Ctrl Pts',(3.51835057975361,33.1281999223435,-1.08074165960988));
#6415=CARTESIAN_POINT('Ctrl Pts',(3.5,33.2531999223435,0.0564772772052952));
#6416=CARTESIAN_POINT('Ctrl Pts',(3.48164942024639,33.3781999223435,1.19369621402047));
#6417=CARTESIAN_POINT('Ctrl Pts',(2.79836296968141,33.5031999223435,2.10293946007876));
#6418=CARTESIAN_POINT('Ctrl Pts',(2.11507651911643,33.6281999223435,3.01218270613706));
#6419=CARTESIAN_POINT('Ctrl Pts',(1.02784639780361,33.7531999223435,3.3461502454855));
#6420=CARTESIAN_POINT('Ctrl Pts',(-0.0593837235092006,33.8781999223435,
3.68011778483394));
#6421=CARTESIAN_POINT('Ctrl Pts',(-1.13527256282102,34.0031999223435,3.31124536858058));
#6422=CARTESIAN_POINT('Ctrl Pts',(-2.21116140213284,34.1281999223436,2.94237295232722));
#6423=CARTESIAN_POINT('Ctrl Pts',(-2.86475599094322,34.2531999223436,2.01155730596855));
#6424=CARTESIAN_POINT('Ctrl Pts',(-3.51835057975361,34.3781999223435,1.08074165960988));
#6425=CARTESIAN_POINT('Ctrl Pts',(-3.5,34.5031999223435,-0.0564772772052956));
#6426=CARTESIAN_POINT('Ctrl Pts',(-3.48164942024639,34.6281999223435,-1.19369621402047));
#6427=CARTESIAN_POINT('Ctrl Pts',(-2.79836296968141,34.7531999223435,-2.10293946007877));
#6428=CARTESIAN_POINT('Ctrl Pts',(-2.11507651911643,34.8781999223436,-3.01218270613706));
#6429=CARTESIAN_POINT('Ctrl Pts',(-1.02784639780361,35.0031999223435,-3.3461502454855));
#6430=CARTESIAN_POINT('Ctrl Pts',(0.0593837235092011,35.1281999223435,-3.68011778483394));
#6431=CARTESIAN_POINT('Ctrl Pts',(1.13527256282102,35.2531999223435,-3.31124536858058));
#6432=CARTESIAN_POINT('Ctrl Pts',(2.21116140213284,35.3781999223435,-2.94237295232722));
#6433=CARTESIAN_POINT('Ctrl Pts',(2.86475599094322,35.5031999223436,-2.01155730596855));
#6434=CARTESIAN_POINT('Ctrl Pts',(3.51835057975361,35.6281999223435,-1.08074165960988));
#6435=CARTESIAN_POINT('Ctrl Pts',(3.5,35.7531999223435,0.0564772772052952));
#6436=CARTESIAN_POINT('Ctrl Pts',(3.48164942024639,35.8781999223435,1.19369621402047));
#6437=CARTESIAN_POINT('Ctrl Pts',(2.79836296968141,36.0031999223435,2.10293946007876));
#6438=CARTESIAN_POINT('Ctrl Pts',(2.11507651911643,36.1281999223436,3.01218270613706));
#6439=CARTESIAN_POINT('Ctrl Pts',(1.02784639780361,36.2531999223435,3.3461502454855));
#6440=CARTESIAN_POINT('Ctrl Pts',(-0.0593837235092006,36.3781999223436,
3.68011778483394));
#6441=CARTESIAN_POINT('Ctrl Pts',(-1.13527256282102,36.5031999223435,3.31124536858058));
#6442=CARTESIAN_POINT('Ctrl Pts',(-2.21116140213284,36.6281999223435,2.94237295232722));
#6443=CARTESIAN_POINT('Ctrl Pts',(-2.86475599094322,36.7531999223435,2.01155730596855));
#6444=CARTESIAN_POINT('Ctrl Pts',(-3.51835057975361,36.8781999223435,1.08074165960988));
#6445=CARTESIAN_POINT('Ctrl Pts',(-3.5,37.0031999223435,-0.0564772772052956));
#6446=CARTESIAN_POINT('Ctrl Pts',(-3.48164942024639,37.1281999223435,-1.19369621402047));
#6447=CARTESIAN_POINT('Ctrl Pts',(-2.79836296968141,37.2531999223435,-2.10293946007877));
#6448=CARTESIAN_POINT('Ctrl Pts',(-2.11507651911643,37.3781999223435,-3.01218270613706));
#6449=CARTESIAN_POINT('Ctrl Pts',(-1.02784639780361,37.5031999223435,-3.3461502454855));
#6450=CARTESIAN_POINT('Ctrl Pts',(0.0593837235092011,37.6281999223435,-3.68011778483394));
#6451=CARTESIAN_POINT('Ctrl Pts',(1.13527256282102,37.7531999223435,-3.31124536858058));
#6452=CARTESIAN_POINT('Ctrl Pts',(2.21116140213284,37.8781999223435,-2.94237295232722));
#6453=CARTESIAN_POINT('Ctrl Pts',(2.86475599094322,38.0031999223435,-2.01155730596855));
#6454=CARTESIAN_POINT('Ctrl Pts',(3.51835057975361,38.1281999223435,-1.08074165960988));
#6455=CARTESIAN_POINT('Ctrl Pts',(3.5,38.2531999223435,0.0564772772052952));
#6456=CARTESIAN_POINT('Ctrl Pts',(3.48164942024639,38.3781999223435,1.19369621402047));
#6457=CARTESIAN_POINT('Ctrl Pts',(2.79836296968141,38.5031999223435,2.10293946007876));
#6458=CARTESIAN_POINT('Ctrl Pts',(2.11507651911643,38.6281999223436,3.01218270613706));
#6459=CARTESIAN_POINT('Ctrl Pts',(1.02784639780361,38.7531999223435,3.3461502454855));
#6460=CARTESIAN_POINT('Ctrl Pts',(-0.0593837235092006,38.8781999223435,
3.68011778483394));
#6461=CARTESIAN_POINT('Ctrl Pts',(-1.13527256282102,39.0031999223435,3.31124536858058));
#6462=CARTESIAN_POINT('Ctrl Pts',(-2.21116140213284,39.1281999223435,2.94237295232722));
#6463=CARTESIAN_POINT('Ctrl Pts',(-2.86475599094322,39.2531999223436,2.01155730596855));
#6464=CARTESIAN_POINT('Ctrl Pts',(-3.51835057975361,39.3781999223435,1.08074165960988));
#6465=CARTESIAN_POINT('Ctrl Pts',(-3.5,39.5031999223435,-0.0564772772052956));
#6466=CARTESIAN_POINT('Ctrl Pts',(-4.5,14.5031999223435,-0.0564772772052853));
#6467=CARTESIAN_POINT('Ctrl Pts',(-4.4816494202464,14.6281999223435,-1.51861591025336));
#6468=CARTESIAN_POINT('Ctrl Pts',(-3.60737996405636,14.7531999223435,-2.69072471237123));
#6469=CARTESIAN_POINT('Ctrl Pts',(-2.73311050786633,14.8781999223435,-3.8628335144891));
#6470=CARTESIAN_POINT('Ctrl Pts',(-1.33686339217857,15.0031999223435,-4.29720676178065));
#6471=CARTESIAN_POINT('Ctrl Pts',(0.0593837235091902,15.1281999223435,-4.7315800090722));
#6472=CARTESIAN_POINT('Ctrl Pts',(1.44428955719596,15.2531999223435,-4.26230188487573));
#6473=CARTESIAN_POINT('Ctrl Pts',(2.82919539088272,15.3781999223435,-3.79302376067926));
#6474=CARTESIAN_POINT('Ctrl Pts',(3.67377298531816,15.5031999223435,-2.59934255826103));
#6475=CARTESIAN_POINT('Ctrl Pts',(4.5183505797536,15.6281999223435,-1.40566135584279));
#6476=CARTESIAN_POINT('Ctrl Pts',(4.5,15.7531999223435,0.0564772772052848));
#6477=CARTESIAN_POINT('Ctrl Pts',(4.4816494202464,15.8781999223435,1.51861591025336));
#6478=CARTESIAN_POINT('Ctrl Pts',(3.60737996405636,16.0031999223435,2.69072471237123));
#6479=CARTESIAN_POINT('Ctrl Pts',(2.73311050786633,16.1281999223435,3.8628335144891));
#6480=CARTESIAN_POINT('Ctrl Pts',(1.33686339217857,16.2531999223435,4.29720676178065));
#6481=CARTESIAN_POINT('Ctrl Pts',(-0.0593837235091896,16.3781999223435,
4.7315800090722));
#6482=CARTESIAN_POINT('Ctrl Pts',(-1.44428955719596,16.5031999223435,4.26230188487573));
#6483=CARTESIAN_POINT('Ctrl Pts',(-2.82919539088272,16.6281999223435,3.79302376067927));
#6484=CARTESIAN_POINT('Ctrl Pts',(-3.67377298531816,16.7531999223435,2.59934255826103));
#6485=CARTESIAN_POINT('Ctrl Pts',(-4.5183505797536,16.8781999223435,1.40566135584279));
#6486=CARTESIAN_POINT('Ctrl Pts',(-4.5,17.0031999223435,-0.0564772772052853));
#6487=CARTESIAN_POINT('Ctrl Pts',(-4.4816494202464,17.1281999223435,-1.51861591025336));
#6488=CARTESIAN_POINT('Ctrl Pts',(-3.60737996405636,17.2531999223435,-2.69072471237123));
#6489=CARTESIAN_POINT('Ctrl Pts',(-2.73311050786633,17.3781999223435,-3.8628335144891));
#6490=CARTESIAN_POINT('Ctrl Pts',(-1.33686339217857,17.5031999223435,-4.29720676178065));
#6491=CARTESIAN_POINT('Ctrl Pts',(0.0593837235091902,17.6281999223435,-4.7315800090722));
#6492=CARTESIAN_POINT('Ctrl Pts',(1.44428955719596,17.7531999223435,-4.26230188487573));
#6493=CARTESIAN_POINT('Ctrl Pts',(2.82919539088272,17.8781999223435,-3.79302376067926));
#6494=CARTESIAN_POINT('Ctrl Pts',(3.67377298531816,18.0031999223435,-2.59934255826103));
#6495=CARTESIAN_POINT('Ctrl Pts',(4.5183505797536,18.1281999223435,-1.40566135584279));
#6496=CARTESIAN_POINT('Ctrl Pts',(4.5,18.2531999223435,0.0564772772052848));
#6497=CARTESIAN_POINT('Ctrl Pts',(4.4816494202464,18.3781999223435,1.51861591025336));
#6498=CARTESIAN_POINT('Ctrl Pts',(3.60737996405636,18.5031999223435,2.69072471237123));
#6499=CARTESIAN_POINT('Ctrl Pts',(2.73311050786633,18.6281999223435,3.8628335144891));
#6500=CARTESIAN_POINT('Ctrl Pts',(1.33686339217857,18.7531999223435,4.29720676178065));
#6501=CARTESIAN_POINT('Ctrl Pts',(-0.0593837235091896,18.8781999223435,
4.7315800090722));
#6502=CARTESIAN_POINT('Ctrl Pts',(-1.44428955719596,19.0031999223435,4.26230188487573));
#6503=CARTESIAN_POINT('Ctrl Pts',(-2.82919539088272,19.1281999223435,3.79302376067927));
#6504=CARTESIAN_POINT('Ctrl Pts',(-3.67377298531816,19.2531999223435,2.59934255826103));
#6505=CARTESIAN_POINT('Ctrl Pts',(-4.5183505797536,19.3781999223435,1.40566135584279));
#6506=CARTESIAN_POINT('Ctrl Pts',(-4.5,19.5031999223435,-0.0564772772052853));
#6507=CARTESIAN_POINT('Ctrl Pts',(-4.4816494202464,19.6281999223435,-1.51861591025336));
#6508=CARTESIAN_POINT('Ctrl Pts',(-3.60737996405636,19.7531999223435,-2.69072471237123));
#6509=CARTESIAN_POINT('Ctrl Pts',(-2.73311050786633,19.8781999223435,-3.8628335144891));
#6510=CARTESIAN_POINT('Ctrl Pts',(-1.33686339217857,20.0031999223435,-4.29720676178065));
#6511=CARTESIAN_POINT('Ctrl Pts',(0.0593837235091902,20.1281999223435,-4.7315800090722));
#6512=CARTESIAN_POINT('Ctrl Pts',(1.44428955719596,20.2531999223435,-4.26230188487573));
#6513=CARTESIAN_POINT('Ctrl Pts',(2.82919539088272,20.3781999223435,-3.79302376067926));
#6514=CARTESIAN_POINT('Ctrl Pts',(3.67377298531816,20.5031999223435,-2.59934255826103));
#6515=CARTESIAN_POINT('Ctrl Pts',(4.5183505797536,20.6281999223435,-1.40566135584279));
#6516=CARTESIAN_POINT('Ctrl Pts',(4.5,20.7531999223435,0.0564772772052848));
#6517=CARTESIAN_POINT('Ctrl Pts',(4.4816494202464,20.8781999223435,1.51861591025336));
#6518=CARTESIAN_POINT('Ctrl Pts',(3.60737996405636,21.0031999223435,2.69072471237123));
#6519=CARTESIAN_POINT('Ctrl Pts',(2.73311050786633,21.1281999223435,3.8628335144891));
#6520=CARTESIAN_POINT('Ctrl Pts',(1.33686339217857,21.2531999223435,4.29720676178065));
#6521=CARTESIAN_POINT('Ctrl Pts',(-0.0593837235091896,21.3781999223435,
4.7315800090722));
#6522=CARTESIAN_POINT('Ctrl Pts',(-1.44428955719596,21.5031999223435,4.26230188487573));
#6523=CARTESIAN_POINT('Ctrl Pts',(-2.82919539088272,21.6281999223435,3.79302376067927));
#6524=CARTESIAN_POINT('Ctrl Pts',(-3.67377298531816,21.7531999223435,2.59934255826103));
#6525=CARTESIAN_POINT('Ctrl Pts',(-4.5183505797536,21.8781999223435,1.40566135584279));
#6526=CARTESIAN_POINT('Ctrl Pts',(-4.5,22.0031999223435,-0.0564772772052853));
#6527=CARTESIAN_POINT('Ctrl Pts',(-4.4816494202464,22.1281999223435,-1.51861591025336));
#6528=CARTESIAN_POINT('Ctrl Pts',(-3.60737996405636,22.2531999223435,-2.69072471237123));
#6529=CARTESIAN_POINT('Ctrl Pts',(-2.73311050786633,22.3781999223435,-3.8628335144891));
#6530=CARTESIAN_POINT('Ctrl Pts',(-1.33686339217857,22.5031999223435,-4.29720676178065));
#6531=CARTESIAN_POINT('Ctrl Pts',(0.0593837235091902,22.6281999223435,-4.7315800090722));
#6532=CARTESIAN_POINT('Ctrl Pts',(1.44428955719596,22.7531999223435,-4.26230188487573));
#6533=CARTESIAN_POINT('Ctrl Pts',(2.82919539088272,22.8781999223435,-3.79302376067926));
#6534=CARTESIAN_POINT('Ctrl Pts',(3.67377298531816,23.0031999223435,-2.59934255826103));
#6535=CARTESIAN_POINT('Ctrl Pts',(4.5183505797536,23.1281999223435,-1.40566135584279));
#6536=CARTESIAN_POINT('Ctrl Pts',(4.5,23.2531999223435,0.0564772772052848));
#6537=CARTESIAN_POINT('Ctrl Pts',(4.4816494202464,23.3781999223435,1.51861591025336));
#6538=CARTESIAN_POINT('Ctrl Pts',(3.60737996405636,23.5031999223435,2.69072471237123));
#6539=CARTESIAN_POINT('Ctrl Pts',(2.73311050786633,23.6281999223435,3.8628335144891));
#6540=CARTESIAN_POINT('Ctrl Pts',(1.33686339217857,23.7531999223435,4.29720676178065));
#6541=CARTESIAN_POINT('Ctrl Pts',(-0.0593837235091896,23.8781999223435,
4.7315800090722));
#6542=CARTESIAN_POINT('Ctrl Pts',(-1.44428955719596,24.0031999223435,4.26230188487573));
#6543=CARTESIAN_POINT('Ctrl Pts',(-2.82919539088272,24.1281999223435,3.79302376067927));
#6544=CARTESIAN_POINT('Ctrl Pts',(-3.67377298531816,24.2531999223435,2.59934255826103));
#6545=CARTESIAN_POINT('Ctrl Pts',(-4.5183505797536,24.3781999223435,1.40566135584279));
#6546=CARTESIAN_POINT('Ctrl Pts',(-4.5,24.5031999223436,-0.0564772772052853));
#6547=CARTESIAN_POINT('Ctrl Pts',(-4.4816494202464,24.6281999223435,-1.51861591025336));
#6548=CARTESIAN_POINT('Ctrl Pts',(-3.60737996405636,24.7531999223435,-2.69072471237123));
#6549=CARTESIAN_POINT('Ctrl Pts',(-2.73311050786633,24.8781999223436,-3.8628335144891));
#6550=CARTESIAN_POINT('Ctrl Pts',(-1.33686339217857,25.0031999223435,-4.29720676178065));
#6551=CARTESIAN_POINT('Ctrl Pts',(0.0593837235091902,25.1281999223435,-4.7315800090722));
#6552=CARTESIAN_POINT('Ctrl Pts',(1.44428955719596,25.2531999223435,-4.26230188487573));
#6553=CARTESIAN_POINT('Ctrl Pts',(2.82919539088272,25.3781999223435,-3.79302376067926));
#6554=CARTESIAN_POINT('Ctrl Pts',(3.67377298531816,25.5031999223435,-2.59934255826103));
#6555=CARTESIAN_POINT('Ctrl Pts',(4.5183505797536,25.6281999223435,-1.40566135584279));
#6556=CARTESIAN_POINT('Ctrl Pts',(4.5,25.7531999223436,0.0564772772052848));
#6557=CARTESIAN_POINT('Ctrl Pts',(4.4816494202464,25.8781999223436,1.51861591025336));
#6558=CARTESIAN_POINT('Ctrl Pts',(3.60737996405636,26.0031999223435,2.69072471237123));
#6559=CARTESIAN_POINT('Ctrl Pts',(2.73311050786633,26.1281999223435,3.8628335144891));
#6560=CARTESIAN_POINT('Ctrl Pts',(1.33686339217857,26.2531999223435,4.29720676178065));
#6561=CARTESIAN_POINT('Ctrl Pts',(-0.0593837235091896,26.3781999223436,
4.7315800090722));
#6562=CARTESIAN_POINT('Ctrl Pts',(-1.44428955719596,26.5031999223435,4.26230188487573));
#6563=CARTESIAN_POINT('Ctrl Pts',(-2.82919539088272,26.6281999223435,3.79302376067927));
#6564=CARTESIAN_POINT('Ctrl Pts',(-3.67377298531816,26.7531999223436,2.59934255826103));
#6565=CARTESIAN_POINT('Ctrl Pts',(-4.5183505797536,26.8781999223435,1.40566135584279));
#6566=CARTESIAN_POINT('Ctrl Pts',(-4.5,27.0031999223436,-0.0564772772052853));
#6567=CARTESIAN_POINT('Ctrl Pts',(-4.4816494202464,27.1281999223436,-1.51861591025336));
#6568=CARTESIAN_POINT('Ctrl Pts',(-3.60737996405636,27.2531999223435,-2.69072471237123));
#6569=CARTESIAN_POINT('Ctrl Pts',(-2.73311050786633,27.3781999223436,-3.8628335144891));
#6570=CARTESIAN_POINT('Ctrl Pts',(-1.33686339217857,27.5031999223435,-4.29720676178065));
#6571=CARTESIAN_POINT('Ctrl Pts',(0.0593837235091902,27.6281999223435,-4.7315800090722));
#6572=CARTESIAN_POINT('Ctrl Pts',(1.44428955719596,27.7531999223435,-4.26230188487573));
#6573=CARTESIAN_POINT('Ctrl Pts',(2.82919539088272,27.8781999223435,-3.79302376067926));
#6574=CARTESIAN_POINT('Ctrl Pts',(3.67377298531816,28.0031999223436,-2.59934255826103));
#6575=CARTESIAN_POINT('Ctrl Pts',(4.5183505797536,28.1281999223435,-1.40566135584279));
#6576=CARTESIAN_POINT('Ctrl Pts',(4.5,28.2531999223435,0.0564772772052848));
#6577=CARTESIAN_POINT('Ctrl Pts',(4.4816494202464,28.3781999223436,1.51861591025336));
#6578=CARTESIAN_POINT('Ctrl Pts',(3.60737996405636,28.5031999223435,2.69072471237123));
#6579=CARTESIAN_POINT('Ctrl Pts',(2.73311050786633,28.6281999223435,3.8628335144891));
#6580=CARTESIAN_POINT('Ctrl Pts',(1.33686339217857,28.7531999223435,4.29720676178065));
#6581=CARTESIAN_POINT('Ctrl Pts',(-0.0593837235091896,28.8781999223435,
4.7315800090722));
#6582=CARTESIAN_POINT('Ctrl Pts',(-1.44428955719596,29.0031999223435,4.26230188487573));
#6583=CARTESIAN_POINT('Ctrl Pts',(-2.82919539088272,29.1281999223435,3.79302376067927));
#6584=CARTESIAN_POINT('Ctrl Pts',(-3.67377298531816,29.2531999223435,2.59934255826103));
#6585=CARTESIAN_POINT('Ctrl Pts',(-4.5183505797536,29.3781999223436,1.40566135584279));
#6586=CARTESIAN_POINT('Ctrl Pts',(-4.5,29.5031999223435,-0.0564772772052853));
#6587=CARTESIAN_POINT('Ctrl Pts',(-4.4816494202464,29.6281999223435,-1.51861591025336));
#6588=CARTESIAN_POINT('Ctrl Pts',(-3.60737996405636,29.7531999223435,-2.69072471237123));
#6589=CARTESIAN_POINT('Ctrl Pts',(-2.73311050786633,29.8781999223435,-3.8628335144891));
#6590=CARTESIAN_POINT('Ctrl Pts',(-1.33686339217857,30.0031999223435,-4.29720676178065));
#6591=CARTESIAN_POINT('Ctrl Pts',(0.0593837235091902,30.1281999223435,-4.7315800090722));
#6592=CARTESIAN_POINT('Ctrl Pts',(1.44428955719596,30.2531999223435,-4.26230188487573));
#6593=CARTESIAN_POINT('Ctrl Pts',(2.82919539088272,30.3781999223435,-3.79302376067926));
#6594=CARTESIAN_POINT('Ctrl Pts',(3.67377298531816,30.5031999223435,-2.59934255826103));
#6595=CARTESIAN_POINT('Ctrl Pts',(4.5183505797536,30.6281999223435,-1.40566135584279));
#6596=CARTESIAN_POINT('Ctrl Pts',(4.5,30.7531999223435,0.0564772772052848));
#6597=CARTESIAN_POINT('Ctrl Pts',(4.4816494202464,30.8781999223435,1.51861591025336));
#6598=CARTESIAN_POINT('Ctrl Pts',(3.60737996405636,31.0031999223435,2.69072471237123));
#6599=CARTESIAN_POINT('Ctrl Pts',(2.73311050786633,31.1281999223435,3.8628335144891));
#6600=CARTESIAN_POINT('Ctrl Pts',(1.33686339217857,31.2531999223435,4.29720676178065));
#6601=CARTESIAN_POINT('Ctrl Pts',(-0.0593837235091896,31.3781999223435,
4.7315800090722));
#6602=CARTESIAN_POINT('Ctrl Pts',(-1.44428955719596,31.5031999223435,4.26230188487573));
#6603=CARTESIAN_POINT('Ctrl Pts',(-2.82919539088272,31.6281999223435,3.79302376067927));
#6604=CARTESIAN_POINT('Ctrl Pts',(-3.67377298531816,31.7531999223436,2.59934255826103));
#6605=CARTESIAN_POINT('Ctrl Pts',(-4.5183505797536,31.8781999223435,1.40566135584279));
#6606=CARTESIAN_POINT('Ctrl Pts',(-4.5,32.0031999223435,-0.0564772772052853));
#6607=CARTESIAN_POINT('Ctrl Pts',(-4.4816494202464,32.1281999223435,-1.51861591025336));
#6608=CARTESIAN_POINT('Ctrl Pts',(-3.60737996405636,32.2531999223435,-2.69072471237123));
#6609=CARTESIAN_POINT('Ctrl Pts',(-2.73311050786633,32.3781999223435,-3.8628335144891));
#6610=CARTESIAN_POINT('Ctrl Pts',(-1.33686339217857,32.5031999223435,-4.29720676178065));
#6611=CARTESIAN_POINT('Ctrl Pts',(0.0593837235091902,32.6281999223435,-4.7315800090722));
#6612=CARTESIAN_POINT('Ctrl Pts',(1.44428955719596,32.7531999223435,-4.26230188487573));
#6613=CARTESIAN_POINT('Ctrl Pts',(2.82919539088272,32.8781999223435,-3.79302376067926));
#6614=CARTESIAN_POINT('Ctrl Pts',(3.67377298531816,33.0031999223436,-2.59934255826103));
#6615=CARTESIAN_POINT('Ctrl Pts',(4.5183505797536,33.1281999223435,-1.40566135584279));
#6616=CARTESIAN_POINT('Ctrl Pts',(4.5,33.2531999223435,0.0564772772052848));
#6617=CARTESIAN_POINT('Ctrl Pts',(4.4816494202464,33.3781999223435,1.51861591025336));
#6618=CARTESIAN_POINT('Ctrl Pts',(3.60737996405636,33.5031999223435,2.69072471237123));
#6619=CARTESIAN_POINT('Ctrl Pts',(2.73311050786633,33.6281999223436,3.8628335144891));
#6620=CARTESIAN_POINT('Ctrl Pts',(1.33686339217857,33.7531999223435,4.29720676178065));
#6621=CARTESIAN_POINT('Ctrl Pts',(-0.0593837235091896,33.8781999223435,
4.7315800090722));
#6622=CARTESIAN_POINT('Ctrl Pts',(-1.44428955719596,34.0031999223435,4.26230188487573));
#6623=CARTESIAN_POINT('Ctrl Pts',(-2.82919539088272,34.1281999223435,3.79302376067927));
#6624=CARTESIAN_POINT('Ctrl Pts',(-3.67377298531816,34.2531999223435,2.59934255826103));
#6625=CARTESIAN_POINT('Ctrl Pts',(-4.5183505797536,34.3781999223435,1.40566135584279));
#6626=CARTESIAN_POINT('Ctrl Pts',(-4.5,34.5031999223435,-0.0564772772052853));
#6627=CARTESIAN_POINT('Ctrl Pts',(-4.4816494202464,34.6281999223435,-1.51861591025336));
#6628=CARTESIAN_POINT('Ctrl Pts',(-3.60737996405636,34.7531999223435,-2.69072471237123));
#6629=CARTESIAN_POINT('Ctrl Pts',(-2.73311050786633,34.8781999223436,-3.8628335144891));
#6630=CARTESIAN_POINT('Ctrl Pts',(-1.33686339217857,35.0031999223435,-4.29720676178065));
#6631=CARTESIAN_POINT('Ctrl Pts',(0.0593837235091902,35.1281999223435,-4.7315800090722));
#6632=CARTESIAN_POINT('Ctrl Pts',(1.44428955719596,35.2531999223435,-4.26230188487573));
#6633=CARTESIAN_POINT('Ctrl Pts',(2.82919539088272,35.3781999223435,-3.79302376067926));
#6634=CARTESIAN_POINT('Ctrl Pts',(3.67377298531816,35.5031999223436,-2.59934255826103));
#6635=CARTESIAN_POINT('Ctrl Pts',(4.5183505797536,35.6281999223435,-1.40566135584279));
#6636=CARTESIAN_POINT('Ctrl Pts',(4.5,35.7531999223435,0.0564772772052848));
#6637=CARTESIAN_POINT('Ctrl Pts',(4.4816494202464,35.8781999223435,1.51861591025336));
#6638=CARTESIAN_POINT('Ctrl Pts',(3.60737996405636,36.0031999223435,2.69072471237123));
#6639=CARTESIAN_POINT('Ctrl Pts',(2.73311050786633,36.1281999223436,3.8628335144891));
#6640=CARTESIAN_POINT('Ctrl Pts',(1.33686339217857,36.2531999223435,4.29720676178065));
#6641=CARTESIAN_POINT('Ctrl Pts',(-0.0593837235091896,36.3781999223435,
4.7315800090722));
#6642=CARTESIAN_POINT('Ctrl Pts',(-1.44428955719596,36.5031999223435,4.26230188487573));
#6643=CARTESIAN_POINT('Ctrl Pts',(-2.82919539088272,36.6281999223435,3.79302376067927));
#6644=CARTESIAN_POINT('Ctrl Pts',(-3.67377298531816,36.7531999223435,2.59934255826103));
#6645=CARTESIAN_POINT('Ctrl Pts',(-4.5183505797536,36.8781999223435,1.40566135584279));
#6646=CARTESIAN_POINT('Ctrl Pts',(-4.5,37.0031999223435,-0.0564772772052853));
#6647=CARTESIAN_POINT('Ctrl Pts',(-4.4816494202464,37.1281999223435,-1.51861591025336));
#6648=CARTESIAN_POINT('Ctrl Pts',(-3.60737996405636,37.2531999223435,-2.69072471237123));
#6649=CARTESIAN_POINT('Ctrl Pts',(-2.73311050786633,37.3781999223436,-3.8628335144891));
#6650=CARTESIAN_POINT('Ctrl Pts',(-1.33686339217857,37.5031999223435,-4.29720676178065));
#6651=CARTESIAN_POINT('Ctrl Pts',(0.0593837235091902,37.6281999223435,-4.7315800090722));
#6652=CARTESIAN_POINT('Ctrl Pts',(1.44428955719596,37.7531999223435,-4.26230188487573));
#6653=CARTESIAN_POINT('Ctrl Pts',(2.82919539088272,37.8781999223435,-3.79302376067926));
#6654=CARTESIAN_POINT('Ctrl Pts',(3.67377298531816,38.0031999223435,-2.59934255826103));
#6655=CARTESIAN_POINT('Ctrl Pts',(4.5183505797536,38.1281999223435,-1.40566135584279));
#6656=CARTESIAN_POINT('Ctrl Pts',(4.5,38.2531999223435,0.0564772772052848));
#6657=CARTESIAN_POINT('Ctrl Pts',(4.4816494202464,38.3781999223435,1.51861591025336));
#6658=CARTESIAN_POINT('Ctrl Pts',(3.60737996405636,38.5031999223435,2.69072471237123));
#6659=CARTESIAN_POINT('Ctrl Pts',(2.73311050786633,38.6281999223436,3.8628335144891));
#6660=CARTESIAN_POINT('Ctrl Pts',(1.33686339217857,38.7531999223435,4.29720676178065));
#6661=CARTESIAN_POINT('Ctrl Pts',(-0.0593837235091896,38.8781999223435,
4.7315800090722));
#6662=CARTESIAN_POINT('Ctrl Pts',(-1.44428955719596,39.0031999223435,4.26230188487573));
#6663=CARTESIAN_POINT('Ctrl Pts',(-2.82919539088272,39.1281999223435,3.79302376067927));
#6664=CARTESIAN_POINT('Ctrl Pts',(-3.67377298531816,39.2531999223436,2.59934255826103));
#6665=CARTESIAN_POINT('Ctrl Pts',(-4.5183505797536,39.3781999223435,1.40566135584279));
#6666=CARTESIAN_POINT('Ctrl Pts',(-4.5,39.5031999223435,-0.0564772772052853));
#6667=CARTESIAN_POINT('Ctrl Pts',(-4.5,15.4968000776565,0.0564772772053793));
#6668=CARTESIAN_POINT('Ctrl Pts',(-4.51835057975363,15.6218000776565,-1.4056613558427));
#6669=CARTESIAN_POINT('Ctrl Pts',(-3.67377298531822,15.7468000776565,-2.59934255826095));
#6670=CARTESIAN_POINT('Ctrl Pts',(-2.82919539088281,15.8718000776565,-3.79302376067921));
#6671=CARTESIAN_POINT('Ctrl Pts',(-1.44428955719605,15.9968000776565,-4.2623018848757));
#6672=CARTESIAN_POINT('Ctrl Pts',(-0.0593837235092896,16.1218000776565,
-4.7315800090722));
#6673=CARTESIAN_POINT('Ctrl Pts',(1.33686339217848,16.2468000776565,-4.29720676178068));
#6674=CARTESIAN_POINT('Ctrl Pts',(2.73311050786625,16.3718000776565,-3.86283351448915));
#6675=CARTESIAN_POINT('Ctrl Pts',(3.60737996405631,16.4968000776565,-2.69072471237131));
#6676=CARTESIAN_POINT('Ctrl Pts',(4.48164942024637,16.6218000776565,-1.51861591025346));
#6677=CARTESIAN_POINT('Ctrl Pts',(4.5,16.7468000776565,-0.0564772772053798));
#6678=CARTESIAN_POINT('Ctrl Pts',(4.51835057975363,16.8718000776565,1.4056613558427));
#6679=CARTESIAN_POINT('Ctrl Pts',(3.67377298531822,16.9968000776565,2.59934255826095));
#6680=CARTESIAN_POINT('Ctrl Pts',(2.82919539088281,17.1218000776565,3.7930237606792));
#6681=CARTESIAN_POINT('Ctrl Pts',(1.44428955719605,17.2468000776565,4.2623018848757));
#6682=CARTESIAN_POINT('Ctrl Pts',(0.0593837235092902,17.3718000776565,4.7315800090722));
#6683=CARTESIAN_POINT('Ctrl Pts',(-1.33686339217848,17.4968000776565,4.29720676178068));
#6684=CARTESIAN_POINT('Ctrl Pts',(-2.73311050786625,17.6218000776565,3.86283351448915));
#6685=CARTESIAN_POINT('Ctrl Pts',(-3.60737996405631,17.7468000776565,2.69072471237131));
#6686=CARTESIAN_POINT('Ctrl Pts',(-4.48164942024637,17.8718000776565,1.51861591025346));
#6687=CARTESIAN_POINT('Ctrl Pts',(-4.5,17.9968000776565,0.0564772772053793));
#6688=CARTESIAN_POINT('Ctrl Pts',(-4.51835057975363,18.1218000776565,-1.4056613558427));
#6689=CARTESIAN_POINT('Ctrl Pts',(-3.67377298531822,18.2468000776565,-2.59934255826095));
#6690=CARTESIAN_POINT('Ctrl Pts',(-2.82919539088281,18.3718000776565,-3.79302376067921));
#6691=CARTESIAN_POINT('Ctrl Pts',(-1.44428955719605,18.4968000776565,-4.2623018848757));
#6692=CARTESIAN_POINT('Ctrl Pts',(-0.0593837235092896,18.6218000776565,
-4.7315800090722));
#6693=CARTESIAN_POINT('Ctrl Pts',(1.33686339217848,18.7468000776565,-4.29720676178068));
#6694=CARTESIAN_POINT('Ctrl Pts',(2.73311050786625,18.8718000776565,-3.86283351448915));
#6695=CARTESIAN_POINT('Ctrl Pts',(3.60737996405631,18.9968000776565,-2.69072471237131));
#6696=CARTESIAN_POINT('Ctrl Pts',(4.48164942024637,19.1218000776565,-1.51861591025346));
#6697=CARTESIAN_POINT('Ctrl Pts',(4.5,19.2468000776565,-0.0564772772053798));
#6698=CARTESIAN_POINT('Ctrl Pts',(4.51835057975363,19.3718000776565,1.4056613558427));
#6699=CARTESIAN_POINT('Ctrl Pts',(3.67377298531822,19.4968000776565,2.59934255826095));
#6700=CARTESIAN_POINT('Ctrl Pts',(2.82919539088281,19.6218000776565,3.7930237606792));
#6701=CARTESIAN_POINT('Ctrl Pts',(1.44428955719605,19.7468000776565,4.2623018848757));
#6702=CARTESIAN_POINT('Ctrl Pts',(0.0593837235092902,19.8718000776565,4.7315800090722));
#6703=CARTESIAN_POINT('Ctrl Pts',(-1.33686339217848,19.9968000776565,4.29720676178068));
#6704=CARTESIAN_POINT('Ctrl Pts',(-2.73311050786625,20.1218000776565,3.86283351448915));
#6705=CARTESIAN_POINT('Ctrl Pts',(-3.60737996405631,20.2468000776565,2.69072471237131));
#6706=CARTESIAN_POINT('Ctrl Pts',(-4.48164942024637,20.3718000776565,1.51861591025346));
#6707=CARTESIAN_POINT('Ctrl Pts',(-4.5,20.4968000776565,0.0564772772053793));
#6708=CARTESIAN_POINT('Ctrl Pts',(-4.51835057975363,20.6218000776565,-1.4056613558427));
#6709=CARTESIAN_POINT('Ctrl Pts',(-3.67377298531822,20.7468000776565,-2.59934255826095));
#6710=CARTESIAN_POINT('Ctrl Pts',(-2.82919539088281,20.8718000776565,-3.79302376067921));
#6711=CARTESIAN_POINT('Ctrl Pts',(-1.44428955719605,20.9968000776565,-4.2623018848757));
#6712=CARTESIAN_POINT('Ctrl Pts',(-0.0593837235092896,21.1218000776565,
-4.7315800090722));
#6713=CARTESIAN_POINT('Ctrl Pts',(1.33686339217848,21.2468000776565,-4.29720676178068));
#6714=CARTESIAN_POINT('Ctrl Pts',(2.73311050786625,21.3718000776565,-3.86283351448915));
#6715=CARTESIAN_POINT('Ctrl Pts',(3.60737996405631,21.4968000776565,-2.69072471237131));
#6716=CARTESIAN_POINT('Ctrl Pts',(4.48164942024637,21.6218000776565,-1.51861591025346));
#6717=CARTESIAN_POINT('Ctrl Pts',(4.5,21.7468000776565,-0.0564772772053798));
#6718=CARTESIAN_POINT('Ctrl Pts',(4.51835057975363,21.8718000776565,1.4056613558427));
#6719=CARTESIAN_POINT('Ctrl Pts',(3.67377298531822,21.9968000776565,2.59934255826095));
#6720=CARTESIAN_POINT('Ctrl Pts',(2.82919539088281,22.1218000776565,3.7930237606792));
#6721=CARTESIAN_POINT('Ctrl Pts',(1.44428955719605,22.2468000776565,4.2623018848757));
#6722=CARTESIAN_POINT('Ctrl Pts',(0.0593837235092902,22.3718000776565,4.7315800090722));
#6723=CARTESIAN_POINT('Ctrl Pts',(-1.33686339217848,22.4968000776565,4.29720676178068));
#6724=CARTESIAN_POINT('Ctrl Pts',(-2.73311050786625,22.6218000776565,3.86283351448915));
#6725=CARTESIAN_POINT('Ctrl Pts',(-3.60737996405631,22.7468000776565,2.69072471237131));
#6726=CARTESIAN_POINT('Ctrl Pts',(-4.48164942024637,22.8718000776565,1.51861591025346));
#6727=CARTESIAN_POINT('Ctrl Pts',(-4.5,22.9968000776565,0.0564772772053793));
#6728=CARTESIAN_POINT('Ctrl Pts',(-4.51835057975363,23.1218000776565,-1.4056613558427));
#6729=CARTESIAN_POINT('Ctrl Pts',(-3.67377298531822,23.2468000776565,-2.59934255826095));
#6730=CARTESIAN_POINT('Ctrl Pts',(-2.82919539088281,23.3718000776565,-3.79302376067921));
#6731=CARTESIAN_POINT('Ctrl Pts',(-1.44428955719605,23.4968000776565,-4.2623018848757));
#6732=CARTESIAN_POINT('Ctrl Pts',(-0.0593837235092896,23.6218000776565,
-4.7315800090722));
#6733=CARTESIAN_POINT('Ctrl Pts',(1.33686339217848,23.7468000776565,-4.29720676178068));
#6734=CARTESIAN_POINT('Ctrl Pts',(2.73311050786625,23.8718000776565,-3.86283351448915));
#6735=CARTESIAN_POINT('Ctrl Pts',(3.60737996405631,23.9968000776565,-2.69072471237131));
#6736=CARTESIAN_POINT('Ctrl Pts',(4.48164942024637,24.1218000776565,-1.51861591025346));
#6737=CARTESIAN_POINT('Ctrl Pts',(4.5,24.2468000776565,-0.0564772772053798));
#6738=CARTESIAN_POINT('Ctrl Pts',(4.51835057975363,24.3718000776565,1.4056613558427));
#6739=CARTESIAN_POINT('Ctrl Pts',(3.67377298531822,24.4968000776565,2.59934255826095));
#6740=CARTESIAN_POINT('Ctrl Pts',(2.82919539088281,24.6218000776565,3.7930237606792));
#6741=CARTESIAN_POINT('Ctrl Pts',(1.44428955719605,24.7468000776565,4.2623018848757));
#6742=CARTESIAN_POINT('Ctrl Pts',(0.0593837235092902,24.8718000776565,4.7315800090722));
#6743=CARTESIAN_POINT('Ctrl Pts',(-1.33686339217848,24.9968000776565,4.29720676178068));
#6744=CARTESIAN_POINT('Ctrl Pts',(-2.73311050786625,25.1218000776565,3.86283351448915));
#6745=CARTESIAN_POINT('Ctrl Pts',(-3.60737996405631,25.2468000776565,2.69072471237131));
#6746=CARTESIAN_POINT('Ctrl Pts',(-4.48164942024637,25.3718000776565,1.51861591025346));
#6747=CARTESIAN_POINT('Ctrl Pts',(-4.5,25.4968000776565,0.0564772772053793));
#6748=CARTESIAN_POINT('Ctrl Pts',(-4.51835057975363,25.6218000776565,-1.4056613558427));
#6749=CARTESIAN_POINT('Ctrl Pts',(-3.67377298531822,25.7468000776565,-2.59934255826095));
#6750=CARTESIAN_POINT('Ctrl Pts',(-2.82919539088281,25.8718000776565,-3.79302376067921));
#6751=CARTESIAN_POINT('Ctrl Pts',(-1.44428955719605,25.9968000776565,-4.2623018848757));
#6752=CARTESIAN_POINT('Ctrl Pts',(-0.0593837235092896,26.1218000776565,
-4.7315800090722));
#6753=CARTESIAN_POINT('Ctrl Pts',(1.33686339217848,26.2468000776565,-4.29720676178068));
#6754=CARTESIAN_POINT('Ctrl Pts',(2.73311050786625,26.3718000776565,-3.86283351448915));
#6755=CARTESIAN_POINT('Ctrl Pts',(3.60737996405631,26.4968000776565,-2.69072471237131));
#6756=CARTESIAN_POINT('Ctrl Pts',(4.48164942024637,26.6218000776565,-1.51861591025346));
#6757=CARTESIAN_POINT('Ctrl Pts',(4.5,26.7468000776565,-0.0564772772053798));
#6758=CARTESIAN_POINT('Ctrl Pts',(4.51835057975363,26.8718000776565,1.4056613558427));
#6759=CARTESIAN_POINT('Ctrl Pts',(3.67377298531822,26.9968000776565,2.59934255826095));
#6760=CARTESIAN_POINT('Ctrl Pts',(2.82919539088281,27.1218000776565,3.7930237606792));
#6761=CARTESIAN_POINT('Ctrl Pts',(1.44428955719605,27.2468000776565,4.2623018848757));
#6762=CARTESIAN_POINT('Ctrl Pts',(0.0593837235092902,27.3718000776565,4.7315800090722));
#6763=CARTESIAN_POINT('Ctrl Pts',(-1.33686339217848,27.4968000776565,4.29720676178068));
#6764=CARTESIAN_POINT('Ctrl Pts',(-2.73311050786625,27.6218000776565,3.86283351448915));
#6765=CARTESIAN_POINT('Ctrl Pts',(-3.60737996405631,27.7468000776565,2.69072471237131));
#6766=CARTESIAN_POINT('Ctrl Pts',(-4.48164942024637,27.8718000776565,1.51861591025346));
#6767=CARTESIAN_POINT('Ctrl Pts',(-4.5,27.9968000776565,0.0564772772053793));
#6768=CARTESIAN_POINT('Ctrl Pts',(-4.51835057975363,28.1218000776565,-1.4056613558427));
#6769=CARTESIAN_POINT('Ctrl Pts',(-3.67377298531822,28.2468000776565,-2.59934255826095));
#6770=CARTESIAN_POINT('Ctrl Pts',(-2.82919539088281,28.3718000776565,-3.79302376067921));
#6771=CARTESIAN_POINT('Ctrl Pts',(-1.44428955719605,28.4968000776565,-4.2623018848757));
#6772=CARTESIAN_POINT('Ctrl Pts',(-0.0593837235092896,28.6218000776565,
-4.7315800090722));
#6773=CARTESIAN_POINT('Ctrl Pts',(1.33686339217848,28.7468000776565,-4.29720676178068));
#6774=CARTESIAN_POINT('Ctrl Pts',(2.73311050786625,28.8718000776565,-3.86283351448915));
#6775=CARTESIAN_POINT('Ctrl Pts',(3.60737996405631,28.9968000776565,-2.69072471237131));
#6776=CARTESIAN_POINT('Ctrl Pts',(4.48164942024637,29.1218000776565,-1.51861591025346));
#6777=CARTESIAN_POINT('Ctrl Pts',(4.5,29.2468000776565,-0.0564772772053798));
#6778=CARTESIAN_POINT('Ctrl Pts',(4.51835057975363,29.3718000776565,1.4056613558427));
#6779=CARTESIAN_POINT('Ctrl Pts',(3.67377298531822,29.4968000776565,2.59934255826095));
#6780=CARTESIAN_POINT('Ctrl Pts',(2.82919539088281,29.6218000776565,3.7930237606792));
#6781=CARTESIAN_POINT('Ctrl Pts',(1.44428955719605,29.7468000776565,4.2623018848757));
#6782=CARTESIAN_POINT('Ctrl Pts',(0.0593837235092902,29.8718000776565,4.7315800090722));
#6783=CARTESIAN_POINT('Ctrl Pts',(-1.33686339217848,29.9968000776565,4.29720676178068));
#6784=CARTESIAN_POINT('Ctrl Pts',(-2.73311050786625,30.1218000776565,3.86283351448915));
#6785=CARTESIAN_POINT('Ctrl Pts',(-3.60737996405631,30.2468000776565,2.69072471237131));
#6786=CARTESIAN_POINT('Ctrl Pts',(-4.48164942024637,30.3718000776565,1.51861591025346));
#6787=CARTESIAN_POINT('Ctrl Pts',(-4.5,30.4968000776565,0.0564772772053793));
#6788=CARTESIAN_POINT('Ctrl Pts',(-4.51835057975363,30.6218000776565,-1.4056613558427));
#6789=CARTESIAN_POINT('Ctrl Pts',(-3.67377298531822,30.7468000776565,-2.59934255826095));
#6790=CARTESIAN_POINT('Ctrl Pts',(-2.82919539088281,30.8718000776565,-3.79302376067921));
#6791=CARTESIAN_POINT('Ctrl Pts',(-1.44428955719605,30.9968000776565,-4.2623018848757));
#6792=CARTESIAN_POINT('Ctrl Pts',(-0.0593837235092896,31.1218000776565,
-4.7315800090722));
#6793=CARTESIAN_POINT('Ctrl Pts',(1.33686339217848,31.2468000776565,-4.29720676178068));
#6794=CARTESIAN_POINT('Ctrl Pts',(2.73311050786625,31.3718000776565,-3.86283351448915));
#6795=CARTESIAN_POINT('Ctrl Pts',(3.60737996405631,31.4968000776565,-2.69072471237131));
#6796=CARTESIAN_POINT('Ctrl Pts',(4.48164942024637,31.6218000776565,-1.51861591025346));
#6797=CARTESIAN_POINT('Ctrl Pts',(4.5,31.7468000776565,-0.0564772772053798));
#6798=CARTESIAN_POINT('Ctrl Pts',(4.51835057975363,31.8718000776565,1.4056613558427));
#6799=CARTESIAN_POINT('Ctrl Pts',(3.67377298531822,31.9968000776565,2.59934255826095));
#6800=CARTESIAN_POINT('Ctrl Pts',(2.82919539088281,32.1218000776565,3.7930237606792));
#6801=CARTESIAN_POINT('Ctrl Pts',(1.44428955719605,32.2468000776565,4.2623018848757));
#6802=CARTESIAN_POINT('Ctrl Pts',(0.0593837235092902,32.3718000776565,4.7315800090722));
#6803=CARTESIAN_POINT('Ctrl Pts',(-1.33686339217848,32.4968000776565,4.29720676178068));
#6804=CARTESIAN_POINT('Ctrl Pts',(-2.73311050786625,32.6218000776565,3.86283351448915));
#6805=CARTESIAN_POINT('Ctrl Pts',(-3.60737996405631,32.7468000776565,2.69072471237131));
#6806=CARTESIAN_POINT('Ctrl Pts',(-4.48164942024637,32.8718000776565,1.51861591025346));
#6807=CARTESIAN_POINT('Ctrl Pts',(-4.5,32.9968000776565,0.0564772772053793));
#6808=CARTESIAN_POINT('Ctrl Pts',(-4.51835057975363,33.1218000776565,-1.4056613558427));
#6809=CARTESIAN_POINT('Ctrl Pts',(-3.67377298531822,33.2468000776565,-2.59934255826095));
#6810=CARTESIAN_POINT('Ctrl Pts',(-2.82919539088281,33.3718000776565,-3.79302376067921));
#6811=CARTESIAN_POINT('Ctrl Pts',(-1.44428955719605,33.4968000776565,-4.2623018848757));
#6812=CARTESIAN_POINT('Ctrl Pts',(-0.0593837235092896,33.6218000776565,
-4.7315800090722));
#6813=CARTESIAN_POINT('Ctrl Pts',(1.33686339217848,33.7468000776565,-4.29720676178068));
#6814=CARTESIAN_POINT('Ctrl Pts',(2.73311050786625,33.8718000776565,-3.86283351448915));
#6815=CARTESIAN_POINT('Ctrl Pts',(3.60737996405631,33.9968000776565,-2.69072471237131));
#6816=CARTESIAN_POINT('Ctrl Pts',(4.48164942024637,34.1218000776565,-1.51861591025346));
#6817=CARTESIAN_POINT('Ctrl Pts',(4.5,34.2468000776565,-0.0564772772053798));
#6818=CARTESIAN_POINT('Ctrl Pts',(4.51835057975363,34.3718000776565,1.4056613558427));
#6819=CARTESIAN_POINT('Ctrl Pts',(3.67377298531822,34.4968000776565,2.59934255826095));
#6820=CARTESIAN_POINT('Ctrl Pts',(2.82919539088281,34.6218000776565,3.7930237606792));
#6821=CARTESIAN_POINT('Ctrl Pts',(1.44428955719605,34.7468000776565,4.2623018848757));
#6822=CARTESIAN_POINT('Ctrl Pts',(0.0593837235092902,34.8718000776565,4.7315800090722));
#6823=CARTESIAN_POINT('Ctrl Pts',(-1.33686339217848,34.9968000776565,4.29720676178068));
#6824=CARTESIAN_POINT('Ctrl Pts',(-2.73311050786625,35.1218000776565,3.86283351448915));
#6825=CARTESIAN_POINT('Ctrl Pts',(-3.60737996405631,35.2468000776565,2.69072471237131));
#6826=CARTESIAN_POINT('Ctrl Pts',(-4.48164942024637,35.3718000776565,1.51861591025346));
#6827=CARTESIAN_POINT('Ctrl Pts',(-4.5,35.4968000776565,0.0564772772053793));
#6828=CARTESIAN_POINT('Ctrl Pts',(-4.51835057975363,35.6218000776565,-1.4056613558427));
#6829=CARTESIAN_POINT('Ctrl Pts',(-3.67377298531822,35.7468000776565,-2.59934255826095));
#6830=CARTESIAN_POINT('Ctrl Pts',(-2.82919539088281,35.8718000776565,-3.79302376067921));
#6831=CARTESIAN_POINT('Ctrl Pts',(-1.44428955719605,35.9968000776565,-4.2623018848757));
#6832=CARTESIAN_POINT('Ctrl Pts',(-0.0593837235092896,36.1218000776565,
-4.7315800090722));
#6833=CARTESIAN_POINT('Ctrl Pts',(1.33686339217848,36.2468000776565,-4.29720676178068));
#6834=CARTESIAN_POINT('Ctrl Pts',(2.73311050786625,36.3718000776565,-3.86283351448915));
#6835=CARTESIAN_POINT('Ctrl Pts',(3.60737996405631,36.4968000776565,-2.69072471237131));
#6836=CARTESIAN_POINT('Ctrl Pts',(4.48164942024637,36.6218000776565,-1.51861591025346));
#6837=CARTESIAN_POINT('Ctrl Pts',(4.5,36.7468000776565,-0.0564772772053798));
#6838=CARTESIAN_POINT('Ctrl Pts',(4.51835057975363,36.8718000776565,1.4056613558427));
#6839=CARTESIAN_POINT('Ctrl Pts',(3.67377298531822,36.9968000776565,2.59934255826095));
#6840=CARTESIAN_POINT('Ctrl Pts',(2.82919539088281,37.1218000776565,3.7930237606792));
#6841=CARTESIAN_POINT('Ctrl Pts',(1.44428955719605,37.2468000776565,4.2623018848757));
#6842=CARTESIAN_POINT('Ctrl Pts',(0.0593837235092902,37.3718000776565,4.7315800090722));
#6843=CARTESIAN_POINT('Ctrl Pts',(-1.33686339217848,37.4968000776565,4.29720676178068));
#6844=CARTESIAN_POINT('Ctrl Pts',(-2.73311050786625,37.6218000776565,3.86283351448915));
#6845=CARTESIAN_POINT('Ctrl Pts',(-3.60737996405631,37.7468000776565,2.69072471237131));
#6846=CARTESIAN_POINT('Ctrl Pts',(-4.48164942024637,37.8718000776565,1.51861591025346));
#6847=CARTESIAN_POINT('Ctrl Pts',(-4.5,37.9968000776565,0.0564772772053793));
#6848=CARTESIAN_POINT('Ctrl Pts',(-4.51835057975363,38.1218000776565,-1.4056613558427));
#6849=CARTESIAN_POINT('Ctrl Pts',(-3.67377298531822,38.2468000776565,-2.59934255826095));
#6850=CARTESIAN_POINT('Ctrl Pts',(-2.82919539088281,38.3718000776565,-3.79302376067921));
#6851=CARTESIAN_POINT('Ctrl Pts',(-1.44428955719605,38.4968000776565,-4.2623018848757));
#6852=CARTESIAN_POINT('Ctrl Pts',(-0.0593837235092896,38.6218000776565,
-4.7315800090722));
#6853=CARTESIAN_POINT('Ctrl Pts',(1.33686339217848,38.7468000776565,-4.29720676178068));
#6854=CARTESIAN_POINT('Ctrl Pts',(2.73311050786625,38.8718000776565,-3.86283351448915));
#6855=CARTESIAN_POINT('Ctrl Pts',(3.60737996405631,38.9968000776565,-2.69072471237131));
#6856=CARTESIAN_POINT('Ctrl Pts',(4.48164942024637,39.1218000776565,-1.51861591025346));
#6857=CARTESIAN_POINT('Ctrl Pts',(4.5,39.2468000776565,-0.0564772772053798));
#6858=CARTESIAN_POINT('Ctrl Pts',(4.51835057975363,39.3718000776565,1.4056613558427));
#6859=CARTESIAN_POINT('Ctrl Pts',(3.67377298531822,39.4968000776565,2.59934255826095));
#6860=CARTESIAN_POINT('Ctrl Pts',(2.82919539088281,39.6218000776565,3.7930237606792));
#6861=CARTESIAN_POINT('Ctrl Pts',(1.44428955719605,39.7468000776565,4.2623018848757));
#6862=CARTESIAN_POINT('Ctrl Pts',(0.0593837235092902,39.8718000776565,4.7315800090722));
#6863=CARTESIAN_POINT('Ctrl Pts',(-1.33686339217848,39.9968000776565,4.29720676178068));
#6864=CARTESIAN_POINT('Ctrl Pts',(-2.73311050786625,40.1218000776565,3.86283351448915));
#6865=CARTESIAN_POINT('Ctrl Pts',(-3.60737996405631,40.2468000776565,2.69072471237131));
#6866=CARTESIAN_POINT('Ctrl Pts',(-4.48164942024637,40.3718000776565,1.51861591025346));
#6867=CARTESIAN_POINT('Ctrl Pts',(-4.5,40.4968000776565,0.0564772772053793));
#6868=CARTESIAN_POINT('Ctrl Pts',(-3.5,15.4968000776565,0.0564772772053689));
#6869=CARTESIAN_POINT('Ctrl Pts',(-3.51835057975363,15.6218000776565,-1.0807416596098));
#6870=CARTESIAN_POINT('Ctrl Pts',(-2.86475599094327,15.7468000776565,-2.01155730596849));
#6871=CARTESIAN_POINT('Ctrl Pts',(-2.2111614021329,15.8718000776565,-2.94237295232717));
#6872=CARTESIAN_POINT('Ctrl Pts',(-1.13527256282109,15.9968000776565,-3.31124536858055));
#6873=CARTESIAN_POINT('Ctrl Pts',(-0.0593837235092786,16.1218000776565,
-3.68011778483394));
#6874=CARTESIAN_POINT('Ctrl Pts',(1.02784639780354,16.2468000776565,-3.34615024548552));
#6875=CARTESIAN_POINT('Ctrl Pts',(2.11507651911636,16.3718000776565,-3.01218270613711));
#6876=CARTESIAN_POINT('Ctrl Pts',(2.79836296968137,16.4968000776565,-2.10293946007882));
#6877=CARTESIAN_POINT('Ctrl Pts',(3.48164942024637,16.6218000776565,-1.19369621402054));
#6878=CARTESIAN_POINT('Ctrl Pts',(3.5,16.7468000776565,-0.0564772772053694));
#6879=CARTESIAN_POINT('Ctrl Pts',(3.51835057975363,16.8718000776565,1.0807416596098));
#6880=CARTESIAN_POINT('Ctrl Pts',(2.86475599094327,16.9968000776565,2.01155730596849));
#6881=CARTESIAN_POINT('Ctrl Pts',(2.2111614021329,17.1218000776565,2.94237295232717));
#6882=CARTESIAN_POINT('Ctrl Pts',(1.13527256282109,17.2468000776565,3.31124536858055));
#6883=CARTESIAN_POINT('Ctrl Pts',(0.0593837235092791,17.3718000776565,3.68011778483394));
#6884=CARTESIAN_POINT('Ctrl Pts',(-1.02784639780354,17.4968000776565,3.34615024548552));
#6885=CARTESIAN_POINT('Ctrl Pts',(-2.11507651911636,17.6218000776565,3.01218270613711));
#6886=CARTESIAN_POINT('Ctrl Pts',(-2.79836296968137,17.7468000776565,2.10293946007882));
#6887=CARTESIAN_POINT('Ctrl Pts',(-3.48164942024637,17.8718000776565,1.19369621402054));
#6888=CARTESIAN_POINT('Ctrl Pts',(-3.5,17.9968000776565,0.0564772772053689));
#6889=CARTESIAN_POINT('Ctrl Pts',(-3.51835057975363,18.1218000776565,-1.0807416596098));
#6890=CARTESIAN_POINT('Ctrl Pts',(-2.86475599094327,18.2468000776565,-2.01155730596849));
#6891=CARTESIAN_POINT('Ctrl Pts',(-2.2111614021329,18.3718000776565,-2.94237295232717));
#6892=CARTESIAN_POINT('Ctrl Pts',(-1.13527256282109,18.4968000776565,-3.31124536858055));
#6893=CARTESIAN_POINT('Ctrl Pts',(-0.0593837235092786,18.6218000776565,
-3.68011778483394));
#6894=CARTESIAN_POINT('Ctrl Pts',(1.02784639780354,18.7468000776565,-3.34615024548552));
#6895=CARTESIAN_POINT('Ctrl Pts',(2.11507651911636,18.8718000776565,-3.01218270613711));
#6896=CARTESIAN_POINT('Ctrl Pts',(2.79836296968137,18.9968000776565,-2.10293946007882));
#6897=CARTESIAN_POINT('Ctrl Pts',(3.48164942024637,19.1218000776565,-1.19369621402054));
#6898=CARTESIAN_POINT('Ctrl Pts',(3.5,19.2468000776565,-0.0564772772053694));
#6899=CARTESIAN_POINT('Ctrl Pts',(3.51835057975363,19.3718000776565,1.0807416596098));
#6900=CARTESIAN_POINT('Ctrl Pts',(2.86475599094327,19.4968000776565,2.01155730596849));
#6901=CARTESIAN_POINT('Ctrl Pts',(2.2111614021329,19.6218000776565,2.94237295232717));
#6902=CARTESIAN_POINT('Ctrl Pts',(1.13527256282109,19.7468000776565,3.31124536858055));
#6903=CARTESIAN_POINT('Ctrl Pts',(0.0593837235092791,19.8718000776565,3.68011778483394));
#6904=CARTESIAN_POINT('Ctrl Pts',(-1.02784639780354,19.9968000776565,3.34615024548552));
#6905=CARTESIAN_POINT('Ctrl Pts',(-2.11507651911636,20.1218000776565,3.01218270613711));
#6906=CARTESIAN_POINT('Ctrl Pts',(-2.79836296968137,20.2468000776565,2.10293946007882));
#6907=CARTESIAN_POINT('Ctrl Pts',(-3.48164942024637,20.3718000776565,1.19369621402054));
#6908=CARTESIAN_POINT('Ctrl Pts',(-3.5,20.4968000776565,0.0564772772053689));
#6909=CARTESIAN_POINT('Ctrl Pts',(-3.51835057975363,20.6218000776565,-1.0807416596098));
#6910=CARTESIAN_POINT('Ctrl Pts',(-2.86475599094327,20.7468000776565,-2.01155730596849));
#6911=CARTESIAN_POINT('Ctrl Pts',(-2.2111614021329,20.8718000776565,-2.94237295232717));
#6912=CARTESIAN_POINT('Ctrl Pts',(-1.13527256282109,20.9968000776565,-3.31124536858055));
#6913=CARTESIAN_POINT('Ctrl Pts',(-0.0593837235092786,21.1218000776565,
-3.68011778483394));
#6914=CARTESIAN_POINT('Ctrl Pts',(1.02784639780354,21.2468000776565,-3.34615024548552));
#6915=CARTESIAN_POINT('Ctrl Pts',(2.11507651911636,21.3718000776565,-3.01218270613711));
#6916=CARTESIAN_POINT('Ctrl Pts',(2.79836296968137,21.4968000776565,-2.10293946007882));
#6917=CARTESIAN_POINT('Ctrl Pts',(3.48164942024637,21.6218000776565,-1.19369621402054));
#6918=CARTESIAN_POINT('Ctrl Pts',(3.5,21.7468000776565,-0.0564772772053694));
#6919=CARTESIAN_POINT('Ctrl Pts',(3.51835057975363,21.8718000776565,1.0807416596098));
#6920=CARTESIAN_POINT('Ctrl Pts',(2.86475599094327,21.9968000776565,2.01155730596849));
#6921=CARTESIAN_POINT('Ctrl Pts',(2.2111614021329,22.1218000776565,2.94237295232717));
#6922=CARTESIAN_POINT('Ctrl Pts',(1.13527256282109,22.2468000776565,3.31124536858055));
#6923=CARTESIAN_POINT('Ctrl Pts',(0.0593837235092791,22.3718000776565,3.68011778483394));
#6924=CARTESIAN_POINT('Ctrl Pts',(-1.02784639780354,22.4968000776565,3.34615024548552));
#6925=CARTESIAN_POINT('Ctrl Pts',(-2.11507651911636,22.6218000776565,3.01218270613711));
#6926=CARTESIAN_POINT('Ctrl Pts',(-2.79836296968137,22.7468000776565,2.10293946007882));
#6927=CARTESIAN_POINT('Ctrl Pts',(-3.48164942024637,22.8718000776565,1.19369621402054));
#6928=CARTESIAN_POINT('Ctrl Pts',(-3.5,22.9968000776565,0.0564772772053689));
#6929=CARTESIAN_POINT('Ctrl Pts',(-3.51835057975363,23.1218000776565,-1.0807416596098));
#6930=CARTESIAN_POINT('Ctrl Pts',(-2.86475599094327,23.2468000776565,-2.01155730596849));
#6931=CARTESIAN_POINT('Ctrl Pts',(-2.2111614021329,23.3718000776565,-2.94237295232717));
#6932=CARTESIAN_POINT('Ctrl Pts',(-1.13527256282109,23.4968000776565,-3.31124536858055));
#6933=CARTESIAN_POINT('Ctrl Pts',(-0.0593837235092786,23.6218000776565,
-3.68011778483394));
#6934=CARTESIAN_POINT('Ctrl Pts',(1.02784639780354,23.7468000776565,-3.34615024548552));
#6935=CARTESIAN_POINT('Ctrl Pts',(2.11507651911636,23.8718000776565,-3.01218270613711));
#6936=CARTESIAN_POINT('Ctrl Pts',(2.79836296968137,23.9968000776565,-2.10293946007882));
#6937=CARTESIAN_POINT('Ctrl Pts',(3.48164942024637,24.1218000776565,-1.19369621402054));
#6938=CARTESIAN_POINT('Ctrl Pts',(3.5,24.2468000776565,-0.0564772772053694));
#6939=CARTESIAN_POINT('Ctrl Pts',(3.51835057975363,24.3718000776565,1.0807416596098));
#6940=CARTESIAN_POINT('Ctrl Pts',(2.86475599094327,24.4968000776565,2.01155730596849));
#6941=CARTESIAN_POINT('Ctrl Pts',(2.2111614021329,24.6218000776565,2.94237295232717));
#6942=CARTESIAN_POINT('Ctrl Pts',(1.13527256282109,24.7468000776565,3.31124536858055));
#6943=CARTESIAN_POINT('Ctrl Pts',(0.0593837235092791,24.8718000776565,3.68011778483394));
#6944=CARTESIAN_POINT('Ctrl Pts',(-1.02784639780354,24.9968000776565,3.34615024548552));
#6945=CARTESIAN_POINT('Ctrl Pts',(-2.11507651911636,25.1218000776565,3.01218270613711));
#6946=CARTESIAN_POINT('Ctrl Pts',(-2.79836296968137,25.2468000776565,2.10293946007882));
#6947=CARTESIAN_POINT('Ctrl Pts',(-3.48164942024637,25.3718000776565,1.19369621402054));
#6948=CARTESIAN_POINT('Ctrl Pts',(-3.5,25.4968000776565,0.0564772772053689));
#6949=CARTESIAN_POINT('Ctrl Pts',(-3.51835057975363,25.6218000776565,-1.0807416596098));
#6950=CARTESIAN_POINT('Ctrl Pts',(-2.86475599094327,25.7468000776565,-2.01155730596849));
#6951=CARTESIAN_POINT('Ctrl Pts',(-2.2111614021329,25.8718000776565,-2.94237295232717));
#6952=CARTESIAN_POINT('Ctrl Pts',(-1.13527256282109,25.9968000776565,-3.31124536858055));
#6953=CARTESIAN_POINT('Ctrl Pts',(-0.0593837235092786,26.1218000776565,
-3.68011778483394));
#6954=CARTESIAN_POINT('Ctrl Pts',(1.02784639780354,26.2468000776565,-3.34615024548552));
#6955=CARTESIAN_POINT('Ctrl Pts',(2.11507651911636,26.3718000776565,-3.01218270613711));
#6956=CARTESIAN_POINT('Ctrl Pts',(2.79836296968137,26.4968000776565,-2.10293946007882));
#6957=CARTESIAN_POINT('Ctrl Pts',(3.48164942024637,26.6218000776565,-1.19369621402054));
#6958=CARTESIAN_POINT('Ctrl Pts',(3.5,26.7468000776565,-0.0564772772053694));
#6959=CARTESIAN_POINT('Ctrl Pts',(3.51835057975363,26.8718000776565,1.0807416596098));
#6960=CARTESIAN_POINT('Ctrl Pts',(2.86475599094327,26.9968000776565,2.01155730596849));
#6961=CARTESIAN_POINT('Ctrl Pts',(2.2111614021329,27.1218000776565,2.94237295232717));
#6962=CARTESIAN_POINT('Ctrl Pts',(1.13527256282109,27.2468000776565,3.31124536858055));
#6963=CARTESIAN_POINT('Ctrl Pts',(0.0593837235092791,27.3718000776565,3.68011778483394));
#6964=CARTESIAN_POINT('Ctrl Pts',(-1.02784639780354,27.4968000776565,3.34615024548552));
#6965=CARTESIAN_POINT('Ctrl Pts',(-2.11507651911636,27.6218000776565,3.01218270613711));
#6966=CARTESIAN_POINT('Ctrl Pts',(-2.79836296968137,27.7468000776565,2.10293946007882));
#6967=CARTESIAN_POINT('Ctrl Pts',(-3.48164942024637,27.8718000776565,1.19369621402054));
#6968=CARTESIAN_POINT('Ctrl Pts',(-3.5,27.9968000776565,0.0564772772053689));
#6969=CARTESIAN_POINT('Ctrl Pts',(-3.51835057975363,28.1218000776565,-1.0807416596098));
#6970=CARTESIAN_POINT('Ctrl Pts',(-2.86475599094327,28.2468000776565,-2.01155730596849));
#6971=CARTESIAN_POINT('Ctrl Pts',(-2.2111614021329,28.3718000776565,-2.94237295232717));
#6972=CARTESIAN_POINT('Ctrl Pts',(-1.13527256282109,28.4968000776565,-3.31124536858055));
#6973=CARTESIAN_POINT('Ctrl Pts',(-0.0593837235092786,28.6218000776565,
-3.68011778483394));
#6974=CARTESIAN_POINT('Ctrl Pts',(1.02784639780354,28.7468000776565,-3.34615024548552));
#6975=CARTESIAN_POINT('Ctrl Pts',(2.11507651911636,28.8718000776565,-3.01218270613711));
#6976=CARTESIAN_POINT('Ctrl Pts',(2.79836296968137,28.9968000776565,-2.10293946007882));
#6977=CARTESIAN_POINT('Ctrl Pts',(3.48164942024637,29.1218000776565,-1.19369621402054));
#6978=CARTESIAN_POINT('Ctrl Pts',(3.5,29.2468000776565,-0.0564772772053694));
#6979=CARTESIAN_POINT('Ctrl Pts',(3.51835057975363,29.3718000776565,1.0807416596098));
#6980=CARTESIAN_POINT('Ctrl Pts',(2.86475599094327,29.4968000776565,2.01155730596849));
#6981=CARTESIAN_POINT('Ctrl Pts',(2.2111614021329,29.6218000776565,2.94237295232717));
#6982=CARTESIAN_POINT('Ctrl Pts',(1.13527256282109,29.7468000776565,3.31124536858055));
#6983=CARTESIAN_POINT('Ctrl Pts',(0.0593837235092791,29.8718000776565,3.68011778483394));
#6984=CARTESIAN_POINT('Ctrl Pts',(-1.02784639780354,29.9968000776565,3.34615024548552));
#6985=CARTESIAN_POINT('Ctrl Pts',(-2.11507651911636,30.1218000776565,3.01218270613711));
#6986=CARTESIAN_POINT('Ctrl Pts',(-2.79836296968137,30.2468000776565,2.10293946007882));
#6987=CARTESIAN_POINT('Ctrl Pts',(-3.48164942024637,30.3718000776565,1.19369621402054));
#6988=CARTESIAN_POINT('Ctrl Pts',(-3.5,30.4968000776565,0.0564772772053689));
#6989=CARTESIAN_POINT('Ctrl Pts',(-3.51835057975363,30.6218000776565,-1.0807416596098));
#6990=CARTESIAN_POINT('Ctrl Pts',(-2.86475599094327,30.7468000776565,-2.01155730596849));
#6991=CARTESIAN_POINT('Ctrl Pts',(-2.2111614021329,30.8718000776565,-2.94237295232717));
#6992=CARTESIAN_POINT('Ctrl Pts',(-1.13527256282109,30.9968000776565,-3.31124536858055));
#6993=CARTESIAN_POINT('Ctrl Pts',(-0.0593837235092786,31.1218000776565,
-3.68011778483394));
#6994=CARTESIAN_POINT('Ctrl Pts',(1.02784639780354,31.2468000776565,-3.34615024548552));
#6995=CARTESIAN_POINT('Ctrl Pts',(2.11507651911636,31.3718000776565,-3.01218270613711));
#6996=CARTESIAN_POINT('Ctrl Pts',(2.79836296968137,31.4968000776565,-2.10293946007882));
#6997=CARTESIAN_POINT('Ctrl Pts',(3.48164942024637,31.6218000776565,-1.19369621402054));
#6998=CARTESIAN_POINT('Ctrl Pts',(3.5,31.7468000776565,-0.0564772772053694));
#6999=CARTESIAN_POINT('Ctrl Pts',(3.51835057975363,31.8718000776565,1.0807416596098));
#7000=CARTESIAN_POINT('Ctrl Pts',(2.86475599094327,31.9968000776565,2.01155730596849));
#7001=CARTESIAN_POINT('Ctrl Pts',(2.2111614021329,32.1218000776565,2.94237295232717));
#7002=CARTESIAN_POINT('Ctrl Pts',(1.13527256282109,32.2468000776565,3.31124536858055));
#7003=CARTESIAN_POINT('Ctrl Pts',(0.0593837235092791,32.3718000776565,3.68011778483394));
#7004=CARTESIAN_POINT('Ctrl Pts',(-1.02784639780354,32.4968000776565,3.34615024548552));
#7005=CARTESIAN_POINT('Ctrl Pts',(-2.11507651911636,32.6218000776565,3.01218270613711));
#7006=CARTESIAN_POINT('Ctrl Pts',(-2.79836296968137,32.7468000776565,2.10293946007882));
#7007=CARTESIAN_POINT('Ctrl Pts',(-3.48164942024637,32.8718000776565,1.19369621402054));
#7008=CARTESIAN_POINT('Ctrl Pts',(-3.5,32.9968000776565,0.0564772772053689));
#7009=CARTESIAN_POINT('Ctrl Pts',(-3.51835057975363,33.1218000776565,-1.0807416596098));
#7010=CARTESIAN_POINT('Ctrl Pts',(-2.86475599094327,33.2468000776565,-2.01155730596849));
#7011=CARTESIAN_POINT('Ctrl Pts',(-2.2111614021329,33.3718000776565,-2.94237295232717));
#7012=CARTESIAN_POINT('Ctrl Pts',(-1.13527256282109,33.4968000776565,-3.31124536858055));
#7013=CARTESIAN_POINT('Ctrl Pts',(-0.0593837235092786,33.6218000776565,
-3.68011778483394));
#7014=CARTESIAN_POINT('Ctrl Pts',(1.02784639780354,33.7468000776565,-3.34615024548552));
#7015=CARTESIAN_POINT('Ctrl Pts',(2.11507651911636,33.8718000776565,-3.01218270613711));
#7016=CARTESIAN_POINT('Ctrl Pts',(2.79836296968137,33.9968000776565,-2.10293946007882));
#7017=CARTESIAN_POINT('Ctrl Pts',(3.48164942024637,34.1218000776565,-1.19369621402054));
#7018=CARTESIAN_POINT('Ctrl Pts',(3.5,34.2468000776565,-0.0564772772053694));
#7019=CARTESIAN_POINT('Ctrl Pts',(3.51835057975363,34.3718000776565,1.0807416596098));
#7020=CARTESIAN_POINT('Ctrl Pts',(2.86475599094327,34.4968000776565,2.01155730596849));
#7021=CARTESIAN_POINT('Ctrl Pts',(2.2111614021329,34.6218000776565,2.94237295232717));
#7022=CARTESIAN_POINT('Ctrl Pts',(1.13527256282109,34.7468000776565,3.31124536858055));
#7023=CARTESIAN_POINT('Ctrl Pts',(0.0593837235092791,34.8718000776565,3.68011778483394));
#7024=CARTESIAN_POINT('Ctrl Pts',(-1.02784639780354,34.9968000776565,3.34615024548552));
#7025=CARTESIAN_POINT('Ctrl Pts',(-2.11507651911636,35.1218000776565,3.01218270613711));
#7026=CARTESIAN_POINT('Ctrl Pts',(-2.79836296968137,35.2468000776565,2.10293946007882));
#7027=CARTESIAN_POINT('Ctrl Pts',(-3.48164942024637,35.3718000776565,1.19369621402054));
#7028=CARTESIAN_POINT('Ctrl Pts',(-3.5,35.4968000776565,0.0564772772053689));
#7029=CARTESIAN_POINT('Ctrl Pts',(-3.51835057975363,35.6218000776565,-1.0807416596098));
#7030=CARTESIAN_POINT('Ctrl Pts',(-2.86475599094327,35.7468000776565,-2.01155730596849));
#7031=CARTESIAN_POINT('Ctrl Pts',(-2.2111614021329,35.8718000776565,-2.94237295232717));
#7032=CARTESIAN_POINT('Ctrl Pts',(-1.13527256282109,35.9968000776565,-3.31124536858055));
#7033=CARTESIAN_POINT('Ctrl Pts',(-0.0593837235092786,36.1218000776565,
-3.68011778483394));
#7034=CARTESIAN_POINT('Ctrl Pts',(1.02784639780354,36.2468000776565,-3.34615024548552));
#7035=CARTESIAN_POINT('Ctrl Pts',(2.11507651911636,36.3718000776565,-3.01218270613711));
#7036=CARTESIAN_POINT('Ctrl Pts',(2.79836296968137,36.4968000776565,-2.10293946007882));
#7037=CARTESIAN_POINT('Ctrl Pts',(3.48164942024637,36.6218000776565,-1.19369621402054));
#7038=CARTESIAN_POINT('Ctrl Pts',(3.5,36.7468000776565,-0.0564772772053694));
#7039=CARTESIAN_POINT('Ctrl Pts',(3.51835057975363,36.8718000776565,1.0807416596098));
#7040=CARTESIAN_POINT('Ctrl Pts',(2.86475599094327,36.9968000776565,2.01155730596849));
#7041=CARTESIAN_POINT('Ctrl Pts',(2.2111614021329,37.1218000776565,2.94237295232717));
#7042=CARTESIAN_POINT('Ctrl Pts',(1.13527256282109,37.2468000776565,3.31124536858055));
#7043=CARTESIAN_POINT('Ctrl Pts',(0.0593837235092791,37.3718000776565,3.68011778483394));
#7044=CARTESIAN_POINT('Ctrl Pts',(-1.02784639780354,37.4968000776565,3.34615024548552));
#7045=CARTESIAN_POINT('Ctrl Pts',(-2.11507651911636,37.6218000776565,3.01218270613711));
#7046=CARTESIAN_POINT('Ctrl Pts',(-2.79836296968137,37.7468000776565,2.10293946007882));
#7047=CARTESIAN_POINT('Ctrl Pts',(-3.48164942024637,37.8718000776565,1.19369621402054));
#7048=CARTESIAN_POINT('Ctrl Pts',(-3.5,37.9968000776565,0.0564772772053689));
#7049=CARTESIAN_POINT('Ctrl Pts',(-3.51835057975363,38.1218000776565,-1.0807416596098));
#7050=CARTESIAN_POINT('Ctrl Pts',(-2.86475599094327,38.2468000776565,-2.01155730596849));
#7051=CARTESIAN_POINT('Ctrl Pts',(-2.2111614021329,38.3718000776565,-2.94237295232717));
#7052=CARTESIAN_POINT('Ctrl Pts',(-1.13527256282109,38.4968000776565,-3.31124536858055));
#7053=CARTESIAN_POINT('Ctrl Pts',(-0.0593837235092786,38.6218000776565,
-3.68011778483394));
#7054=CARTESIAN_POINT('Ctrl Pts',(1.02784639780354,38.7468000776565,-3.34615024548552));
#7055=CARTESIAN_POINT('Ctrl Pts',(2.11507651911636,38.8718000776565,-3.01218270613711));
#7056=CARTESIAN_POINT('Ctrl Pts',(2.79836296968137,38.9968000776565,-2.10293946007882));
#7057=CARTESIAN_POINT('Ctrl Pts',(3.48164942024637,39.1218000776565,-1.19369621402054));
#7058=CARTESIAN_POINT('Ctrl Pts',(3.5,39.2468000776565,-0.0564772772053694));
#7059=CARTESIAN_POINT('Ctrl Pts',(3.51835057975363,39.3718000776565,1.0807416596098));
#7060=CARTESIAN_POINT('Ctrl Pts',(2.86475599094327,39.4968000776565,2.01155730596849));
#7061=CARTESIAN_POINT('Ctrl Pts',(2.2111614021329,39.6218000776565,2.94237295232717));
#7062=CARTESIAN_POINT('Ctrl Pts',(1.13527256282109,39.7468000776565,3.31124536858055));
#7063=CARTESIAN_POINT('Ctrl Pts',(0.0593837235092791,39.8718000776565,3.68011778483394));
#7064=CARTESIAN_POINT('Ctrl Pts',(-1.02784639780354,39.9968000776565,3.34615024548552));
#7065=CARTESIAN_POINT('Ctrl Pts',(-2.11507651911636,40.1218000776565,3.01218270613711));
#7066=CARTESIAN_POINT('Ctrl Pts',(-2.79836296968137,40.2468000776565,2.10293946007882));
#7067=CARTESIAN_POINT('Ctrl Pts',(-3.48164942024637,40.3718000776565,1.19369621402054));
#7068=CARTESIAN_POINT('Ctrl Pts',(-3.5,40.4968000776565,0.0564772772053689));
#7069=CARTESIAN_POINT('Ctrl Pts',(-4.,15.,4.06619182768964E-14));
#7070=CARTESIAN_POINT('Ctrl Pts',(-4.,15.,-0.440632020643727));
#7071=CARTESIAN_POINT('Ctrl Pts',(-3.92185965933852,15.0000000000976,-0.877629741799447));
#7072=CARTESIAN_POINT('Ctrl Pts',(-3.62979221219699,15.0000000000976,-1.66011634884888));
#7073=CARTESIAN_POINT('Ctrl Pts',(-3.43268623534794,15.,-2.00518450039358));
#7074=CARTESIAN_POINT('Ctrl Pts',(-2.88759998961772,15.,-2.67411379288896));
#7075=CARTESIAN_POINT('Ctrl Pts',(-2.5779848430817,15.,-2.90941676657201));
#7076=CARTESIAN_POINT('Ctrl Pts',(-2.01365919589359,15.,-3.24428371091136));
#7077=CARTESIAN_POINT('Ctrl Pts',(-1.72921866213227,15.,-3.34220683205328));
#7078=CARTESIAN_POINT('Ctrl Pts',(-1.36507732602257,15.,-3.41070229712197));
#7079=CARTESIAN_POINT('Ctrl Pts',(-1.24715486254448,15.,-3.41477569775386));
#7080=CARTESIAN_POINT('Ctrl Pts',(-1.14129294530342,15.,-3.39661359285216));
#7081=CARTESIAN_POINT('Ctrl Pts',(-1.11145580616616,14.9999999999902,-3.38885059559076));
#7082=CARTESIAN_POINT('Ctrl Pts',(-1.08075410559423,14.9999999999902,-3.37025735211956));
#7083=CARTESIAN_POINT('Ctrl Pts',(-1.07322843619766,15.,-3.36443481553715));
#7084=CARTESIAN_POINT('Ctrl Pts',(-1.06203758490191,15.,-3.3514938315438));
#7085=CARTESIAN_POINT('Ctrl Pts',(-1.05807836132249,15.,-3.34489686808688));
#7086=CARTESIAN_POINT('Ctrl Pts',(-1.05560584366885,15.,-3.33749696414134));
#7087=CARTESIAN_POINT('Origin',(0.,15.,0.));
#7610=UNCERTAINTY_MEASURE_WITH_UNIT(LENGTH_MEASURE(0.01),#7628,
'DISTANCE_ACCURACY_VALUE',
'Maximum model space distance between geometric entities at asserted c
onnectivities');
#7616=UNCERTAINTY_MEASURE_WITH_UNIT(LENGTH_MEASURE(0.01),#7628,
'DISTANCE_ACCURACY_VALUE',
'Maximum model space distance between geometric entities at asserted c
onnectivities');
#7621=(
GEOMETRIC_REPRESENTATION_CONTEXT(3)
GLOBAL_UNCERTAINTY_ASSIGNED_CONTEXT((#7610))
GLOBAL_UNIT_ASSIGNED_CONTEXT((#7628,#7630,#7631))
REPRESENTATION_CONTEXT('','3D')
);
#7627=(
GEOMETRIC_REPRESENTATION_CONTEXT(3)
GLOBAL_UNCERTAINTY_ASSIGNED_CONTEXT((#7616))
GLOBAL_UNIT_ASSIGNED_CONTEXT((#7628,#7630,#7631))
REPRESENTATION_CONTEXT('','3D')
);
#7628=(
LENGTH_UNIT()
NAMED_UNIT(*)
SI_UNIT(.MILLI.,.METRE.)
);
#7630=(
NAMED_UNIT(*)
PLANE_ANGLE_UNIT()
SI_UNIT($,.RADIAN.)
);
#7631=(
NAMED_UNIT(*)
SI_UNIT($,.STERADIAN.)
SOLID_ANGLE_UNIT()
);
#7636=SHAPE_DEFINITION_REPRESENTATION(#7646,#7668);
#7646=PRODUCT_DEFINITION_SHAPE('',$,#7679);
#7668=SHAPE_REPRESENTATION('',(#2600),#7621);
#7674=PRODUCT_DEFINITION_CONTEXT('part definition',#7706,'design');
#7679=PRODUCT_DEFINITION('Return Spring','Return Spring',#7689,#7674);
#7689=PRODUCT_DEFINITION_FORMATION('',$,#7712);
#7706=APPLICATION_CONTEXT(
'Core Data for Automotive Mechanical Design Process');
#7707=PRODUCT_CONTEXT('part definition',#7706,'mechanical');
#7712=PRODUCT('Return Spring','Return Spring',$,(#7707));
#7722=PRESENTATION_STYLE_ASSIGNMENT((#7728));
#7728=SURFACE_STYLE_USAGE(.BOTH.,#7734);
#7734=SURFACE_SIDE_STYLE('',(#7740));
#7740=SURFACE_STYLE_FILL_AREA(#7746);
#7746=FILL_AREA_STYLE('Opaque(122,133,145)',(#7752));
#7752=FILL_AREA_STYLE_COLOUR('Opaque(122,133,145)',#7758);
#7758=COLOUR_RGB('Opaque(122,133,145)',0.47843137254902,0.52156862745098,
0.568627450980392);
ENDSEC;
END-ISO-10303-21;
